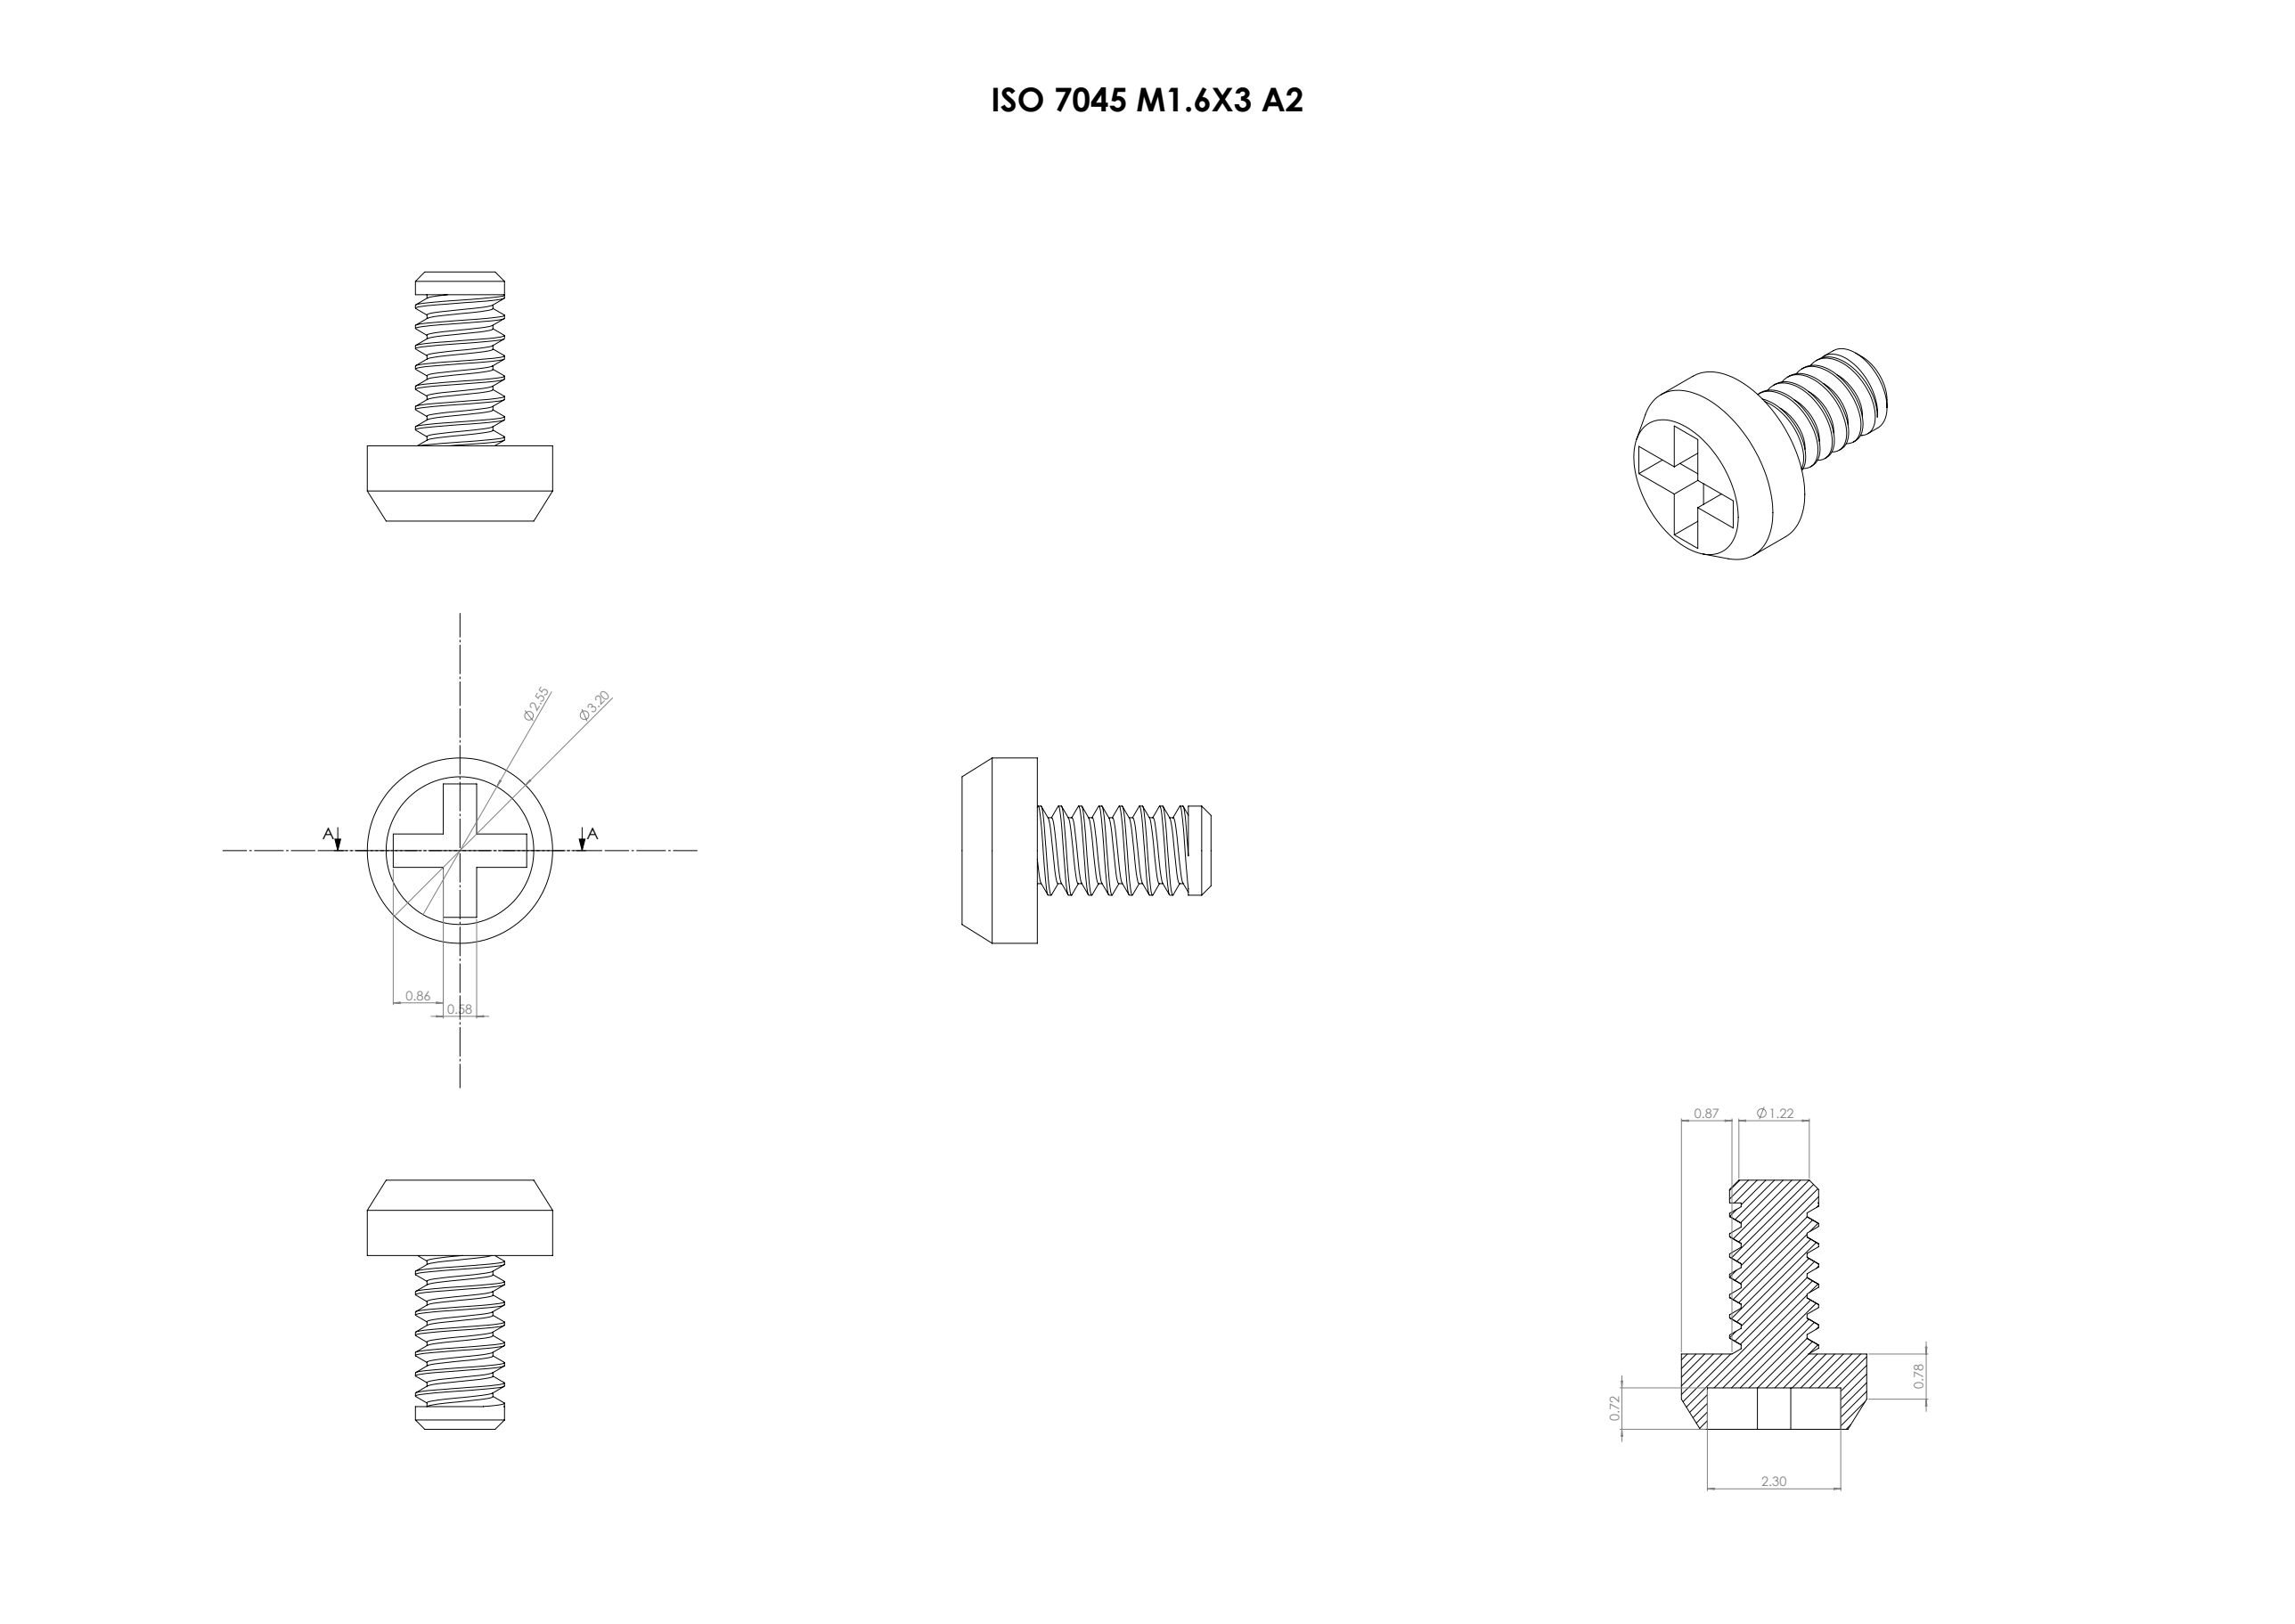
ISO-10303-21;
HEADER;
/* Generated by software containing ST-Developer
 * from STEP Tools, Inc. (www.steptools.com) 
 */

FILE_DESCRIPTION(
/* description */ (''),
/* implementation_level */ '2;1');

FILE_NAME(
/* name */ '18_ISO_7045_M1.6x3_A2.step',
/* time_stamp */ '2026-10-19T23:00:43-07:00',
/* author */ (''),
/* organization */ (''),
/* preprocessor_version */ 'ST-DEVELOPER v20.2',
/* originating_system */ 'Autodesk Translation Framework v15.15.0.0',
/* authorisation */ '');

FILE_SCHEMA (('AUTOMOTIVE_DESIGN { 1 0 10303 214 3 1 1 }'));
ENDSEC;

DATA;
#10=MECHANICAL_DESIGN_GEOMETRIC_PRESENTATION_REPRESENTATION('',(#1014),#55002);
#480=B_SPLINE_SURFACE_WITH_KNOTS('',3,3,((#51812,#51813,#51814,#51815,#51816,
#51817,#51818,#51819,#51820,#51821,#51822,#51823,#51824,#51825,#51826,#51827,
#51828,#51829,#51830,#51831,#51832,#51833,#51834,#51835,#51836,#51837,#51838,
#51839,#51840,#51841,#51842,#51843,#51844,#51845,#51846,#51847,#51848,#51849,
#51850,#51851,#51852,#51853,#51854,#51855,#51856,#51857,#51858,#51859,#51860,
#51861,#51862,#51863),(#51864,#51865,#51866,#51867,#51868,#51869,#51870,
#51871,#51872,#51873,#51874,#51875,#51876,#51877,#51878,#51879,#51880,#51881,
#51882,#51883,#51884,#51885,#51886,#51887,#51888,#51889,#51890,#51891,#51892,
#51893,#51894,#51895,#51896,#51897,#51898,#51899,#51900,#51901,#51902,#51903,
#51904,#51905,#51906,#51907,#51908,#51909,#51910,#51911,#51912,#51913,#51914,
#51915),(#51916,#51917,#51918,#51919,#51920,#51921,#51922,#51923,#51924,
#51925,#51926,#51927,#51928,#51929,#51930,#51931,#51932,#51933,#51934,#51935,
#51936,#51937,#51938,#51939,#51940,#51941,#51942,#51943,#51944,#51945,#51946,
#51947,#51948,#51949,#51950,#51951,#51952,#51953,#51954,#51955,#51956,#51957,
#51958,#51959,#51960,#51961,#51962,#51963,#51964,#51965,#51966,#51967),
(#51968,#51969,#51970,#51971,#51972,#51973,#51974,#51975,#51976,#51977,
#51978,#51979,#51980,#51981,#51982,#51983,#51984,#51985,#51986,#51987,#51988,
#51989,#51990,#51991,#51992,#51993,#51994,#51995,#51996,#51997,#51998,#51999,
#52000,#52001,#52002,#52003,#52004,#52005,#52006,#52007,#52008,#52009,#52010,
#52011,#52012,#52013,#52014,#52015,#52016,#52017,#52018,#52019)),
 .UNSPECIFIED.,.F.,.F.,.F.,(4,4),(4,1,1,1,1,1,1,1,1,1,1,1,1,1,1,1,1,1,1,
1,1,1,1,1,1,1,1,1,1,1,1,1,1,1,1,1,1,1,1,1,1,1,1,1,1,1,1,1,1,4),(0.,0.023094010767585),
(12.4478189520753,13.4456071169044,14.4433952817334,15.4411834465625,16.4389716113915,
17.4367597762206,18.4345479410496,19.4323361058786,20.4301242707077,21.4279124355367,
22.4257006003658,23.4234887651948,24.4212769300238,25.4190650948529,26.4168532596819,
27.414641424511,28.41242958934,29.410217754169,30.4080059189981,31.4057940838271,
32.4035822486562,33.4013704134852,34.3991585783142,35.3969467431433,36.3947349079723,
37.3925230728014,38.3903112376304,39.3880994024594,40.3858875672885,41.3836757321175,
42.3814638969466,43.3792520617756,44.3770402266046,45.3748283914337,46.3726165562627,
47.3704047210918,48.3681928859208,49.3659810507499,50.3637692155789,51.3615573804079,
52.359345545237,53.357133710066,54.3549218748951,55.3527100397241,56.3504982045531,
57.3482863693822,58.3460745342112,59.3438626990403,60.3416508638693,61.3394390286984),
 .UNSPECIFIED.);
#481=B_SPLINE_SURFACE_WITH_KNOTS('',3,3,((#52187,#52188,#52189,#52190,#52191,
#52192,#52193,#52194,#52195,#52196,#52197,#52198,#52199,#52200,#52201,#52202,
#52203,#52204,#52205,#52206,#52207,#52208,#52209,#52210,#52211,#52212,#52213,
#52214,#52215,#52216,#52217,#52218,#52219,#52220,#52221,#52222,#52223,#52224,
#52225,#52226,#52227,#52228,#52229,#52230,#52231,#52232,#52233,#52234,#52235,
#52236,#52237,#52238),(#52239,#52240,#52241,#52242,#52243,#52244,#52245,
#52246,#52247,#52248,#52249,#52250,#52251,#52252,#52253,#52254,#52255,#52256,
#52257,#52258,#52259,#52260,#52261,#52262,#52263,#52264,#52265,#52266,#52267,
#52268,#52269,#52270,#52271,#52272,#52273,#52274,#52275,#52276,#52277,#52278,
#52279,#52280,#52281,#52282,#52283,#52284,#52285,#52286,#52287,#52288,#52289,
#52290),(#52291,#52292,#52293,#52294,#52295,#52296,#52297,#52298,#52299,
#52300,#52301,#52302,#52303,#52304,#52305,#52306,#52307,#52308,#52309,#52310,
#52311,#52312,#52313,#52314,#52315,#52316,#52317,#52318,#52319,#52320,#52321,
#52322,#52323,#52324,#52325,#52326,#52327,#52328,#52329,#52330,#52331,#52332,
#52333,#52334,#52335,#52336,#52337,#52338,#52339,#52340,#52341,#52342),
(#52343,#52344,#52345,#52346,#52347,#52348,#52349,#52350,#52351,#52352,
#52353,#52354,#52355,#52356,#52357,#52358,#52359,#52360,#52361,#52362,#52363,
#52364,#52365,#52366,#52367,#52368,#52369,#52370,#52371,#52372,#52373,#52374,
#52375,#52376,#52377,#52378,#52379,#52380,#52381,#52382,#52383,#52384,#52385,
#52386,#52387,#52388,#52389,#52390,#52391,#52392,#52393,#52394)),
 .UNSPECIFIED.,.F.,.F.,.F.,(4,4),(4,1,1,1,1,1,1,1,1,1,1,1,1,1,1,1,1,1,1,
1,1,1,1,1,1,1,1,1,1,1,1,1,1,1,1,1,1,1,1,1,1,1,1,1,1,1,1,1,1,4),(0.,0.023094010767585),
(15.7552446903951,16.7530328552242,17.7508210200532,18.7486091848822,19.7463973497113,
20.7441855145403,21.7419736793694,22.7397618441984,23.7375500090275,24.7353381738565,
25.7331263386855,26.7309145035146,27.7287026683436,28.7264908331727,29.7242789980017,
30.7220671628307,31.7198553276598,32.7176434924888,33.7154316573179,34.7132198221469,
35.7110079869759,36.708796151805,37.706584316634,38.7043724814631,39.7021606462921,
40.6999488111211,41.6977369759502,42.6955251407792,43.6933133056083,44.6911014704373,
45.6888896352663,46.6866778000954,47.6844659649244,48.6822541297535,49.6800422945825,
50.6778304594116,51.6756186242406,52.6734067890696,53.6711949538987,54.6689831187277,
55.6667712835568,56.6645594483858,57.6623476132148,58.6601357780439,59.6579239428729,
60.655712107702,61.653500272531,62.6512884373601,63.6490766021891,64.6468647670181),
 .UNSPECIFIED.);
#845=B_SPLINE_CURVE_WITH_KNOTS('',3,(#51284,#51285,#51286,#51287,#51288,
#51289,#51290,#51291,#51292,#51293,#51294,#51295,#51296,#51297,#51298,#51299),
 .UNSPECIFIED.,.F.,.F.,(4,3,3,3,3,4),(-6.2359038847334,-5.98672898897424,
-4.9889408241452,-3.99115265931616,-2.99336449448712,-2.07291355912483),
 .UNSPECIFIED.);
#846=B_SPLINE_CURVE_WITH_KNOTS('',3,(#51307,#51308,#51309,#51310,#51311,
#51312,#51313,#51314,#51315,#51316,#51317,#51318,#51319),.UNSPECIFIED.,
 .F.,.F.,(4,3,3,3,4),(0.,0.997788164829036,1.99557632965808,2.99336449448712,
3.26014431587357),.UNSPECIFIED.);
#847=B_SPLINE_CURVE_WITH_KNOTS('',3,(#51324,#51325,#51326,#51327,#51328,
#51329,#51330,#51331,#51332,#51333,#51334,#51335,#51336,#51337,#51338,#51339,
#51340,#51341,#51342,#51343,#51344,#51345),.UNSPECIFIED.,.F.,.F.,(4,3,3,
3,3,3,3,4),(-12.519089191913,-11.9734579779485,-10.9756698131195,-9.97788164829041,
-8.98009348346137,-7.98230531863233,-6.98451715380329,-6.2359038847334),
 .UNSPECIFIED.);
#848=B_SPLINE_CURVE_WITH_KNOTS('',3,(#51346,#51347,#51348,#51349,#51350,
#51351,#51352,#51353,#51354,#51355,#51356,#51357,#51358,#51359,#51360,#51361,
#51362,#51363,#51364,#51365,#51366,#51367),.UNSPECIFIED.,.F.,.F.,(4,3,3,
3,3,3,3,4),(3.26014431587357,3.99115265931617,4.9889408241452,5.98672898897425,
6.98451715380329,7.98230531863232,8.98009348346137,9.54332962305316),
 .UNSPECIFIED.);
#849=B_SPLINE_CURVE_WITH_KNOTS('',3,(#51372,#51373,#51374,#51375,#51376,
#51377,#51378,#51379,#51380,#51381,#51382,#51383,#51384,#51385,#51386,#51387,
#51388,#51389,#51390,#51391,#51392,#51393),.UNSPECIFIED.,.F.,.F.,(4,3,3,
3,3,3,3,4),(-18.8022744990926,-17.9601869669227,-16.9623988020937,-15.9646106372647,
-14.9668224724356,-13.9690343076066,-12.9712461427775,-12.519089191913),
 .UNSPECIFIED.);
#850=B_SPLINE_CURVE_WITH_KNOTS('',3,(#51394,#51395,#51396,#51397,#51398,
#51399,#51400,#51401,#51402,#51403,#51404,#51405,#51406,#51407,#51408,#51409,
#51410,#51411,#51412,#51413,#51414,#51415),.UNSPECIFIED.,.F.,.F.,(4,3,3,
3,3,3,3,4),(9.54332962305316,9.97788164829041,10.9756698131194,11.9734579779485,
12.9712461427775,13.9690343076066,14.9668224724356,15.8265149302327),
 .UNSPECIFIED.);
#851=B_SPLINE_CURVE_WITH_KNOTS('',3,(#51420,#51421,#51422,#51423,#51424,
#51425,#51426,#51427,#51428,#51429,#51430,#51431,#51432,#51433,#51434,#51435,
#51436,#51437,#51438,#51439,#51440,#51441,#51442,#51443,#51444),
 .UNSPECIFIED.,.F.,.F.,(4,3,3,3,3,3,3,3,4),(-25.0854598062722,-24.944704120726,
-23.946915955897,-22.9491277910679,-21.9513396262389,-20.9535514614099,
-19.9557632965808,-18.9579751317518,-18.8022744990926),.UNSPECIFIED.);
#852=B_SPLINE_CURVE_WITH_KNOTS('',3,(#51445,#51446,#51447,#51448,#51449,
#51450,#51451,#51452,#51453,#51454,#51455,#51456,#51457,#51458,#51459,#51460,
#51461,#51462,#51463,#51464,#51465,#51466,#51467,#51468,#51469),
 .UNSPECIFIED.,.F.,.F.,(4,3,3,3,3,3,3,3,4),(15.8265149302327,15.9646106372647,
16.9623988020937,17.9601869669227,18.9579751317518,19.9557632965808,20.9535514614099,
21.9513396262389,22.1097002374123),.UNSPECIFIED.);
#853=B_SPLINE_CURVE_WITH_KNOTS('',3,(#51474,#51475,#51476,#51477,#51478,
#51479,#51480,#51481,#51482,#51483,#51484,#51485,#51486,#51487,#51488,#51489,
#51490,#51491,#51492,#51493,#51494,#51495),.UNSPECIFIED.,.F.,.F.,(4,3,3,
3,3,3,3,4),(-31.3686451134517,-30.9314331097003,-29.9336449448712,-28.9358567800422,
-27.9380686152131,-26.9402804503841,-25.9424922855551,-25.0854598062722),
 .UNSPECIFIED.);
#854=B_SPLINE_CURVE_WITH_KNOTS('',3,(#51496,#51497,#51498,#51499,#51500,
#51501,#51502,#51503,#51504,#51505,#51506,#51507,#51508,#51509,#51510,#51511,
#51512,#51513,#51514,#51515,#51516,#51517),.UNSPECIFIED.,.F.,.F.,(4,3,3,
3,3,3,3,4),(22.1097002374123,22.9491277910679,23.946915955897,24.944704120726,
25.9424922855551,26.9402804503841,27.9380686152131,28.3928855445919),
 .UNSPECIFIED.);
#855=B_SPLINE_CURVE_WITH_KNOTS('',3,(#51522,#51523,#51524,#51525,#51526,
#51527,#51528,#51529,#51530,#51531,#51532,#51533,#51534,#51535,#51536,#51537,
#51538,#51539,#51540,#51541,#51542,#51543),.UNSPECIFIED.,.F.,.F.,(4,3,3,
3,3,3,3,4),(-37.6518304206313,-36.9181620986745,-35.9203739338455,-34.9225857690164,
-33.9247976041874,-32.9270094393584,-31.9292212745293,-31.3686451134517),
 .UNSPECIFIED.);
#856=B_SPLINE_CURVE_WITH_KNOTS('',3,(#51544,#51545,#51546,#51547,#51548,
#51549,#51550,#51551,#51552,#51553,#51554,#51555,#51556,#51557,#51558,#51559,
#51560,#51561,#51562,#51563,#51564,#51565),.UNSPECIFIED.,.F.,.F.,(4,3,3,
3,3,3,3,4),(28.3928855445919,28.9358567800422,29.9336449448712,30.9314331097003,
31.9292212745293,32.9270094393584,33.9247976041874,34.6760708517715),
 .UNSPECIFIED.);
#857=B_SPLINE_CURVE_WITH_KNOTS('',3,(#51570,#51571,#51572,#51573,#51574,
#51575,#51576,#51577,#51578,#51579,#51580,#51581,#51582,#51583,#51584,#51585,
#51586,#51587,#51588,#51589,#51590,#51591,#51592,#51593,#51594),
 .UNSPECIFIED.,.F.,.F.,(4,3,3,3,3,3,3,3,4),(-43.9350157278109,-43.9026792524778,
-42.9048910876488,-41.9071029228197,-40.9093147579907,-39.9115265931616,
-38.9137384283326,-37.9159502635036,-37.6518304206313),.UNSPECIFIED.);
#858=B_SPLINE_CURVE_WITH_KNOTS('',3,(#51595,#51596,#51597,#51598,#51599,
#51600,#51601,#51602,#51603,#51604,#51605,#51606,#51607,#51608,#51609,#51610,
#51611,#51612,#51613,#51614,#51615,#51616,#51617,#51618,#51619),
 .UNSPECIFIED.,.F.,.F.,(4,3,3,3,3,3,3,3,4),(34.6760708517715,34.9225857690164,
35.9203739338455,36.9181620986745,37.9159502635036,38.9137384283326,39.9115265931616,
40.9093147579907,40.9592561589511),.UNSPECIFIED.);
#859=B_SPLINE_CURVE_WITH_KNOTS('',3,(#51625,#51626,#51627,#51628,#51629,
#51630),.UNSPECIFIED.,.F.,.F.,(4,1,1,4),(59.6902604182061,60.655712107702,
61.653500272531,62.5739512078933),.UNSPECIFIED.);
#860=B_SPLINE_CURVE_WITH_KNOTS('',3,(#51633,#51634,#51635,#51636,#51637),
 .UNSPECIFIED.,.F.,.F.,(4,1,4),(59.6902604182061,60.3416508638693,61.3394390286984),
 .UNSPECIFIED.);
#861=B_SPLINE_CURVE_WITH_KNOTS('',3,(#51642,#51643,#51644,#51645,#51646,
#51647,#51648,#51649,#51650,#51651,#51652),.UNSPECIFIED.,.F.,.F.,(4,1,1,
1,1,1,1,1,4),(53.4070751110265,53.6711949538987,54.6689831187277,55.6667712835568,
56.6645594483858,57.6623476132148,58.6601357780439,59.6579239428729,59.6902604182061),
 .UNSPECIFIED.);
#862=B_SPLINE_CURVE_WITH_KNOTS('',3,(#51653,#51654,#51655,#51656,#51657,
#51658,#51659,#51660,#51661,#51662),.UNSPECIFIED.,.F.,.F.,(4,1,1,1,1,1,
1,4),(53.4070751110265,54.3549218748951,55.3527100397241,56.3504982045531,
57.3482863693822,58.3460745342112,59.3438626990403,59.6902604182061),
 .UNSPECIFIED.);
#863=B_SPLINE_CURVE_WITH_KNOTS('',3,(#51667,#51668,#51669,#51670,#51671,
#51672,#51673,#51674,#51675,#51676),.UNSPECIFIED.,.F.,.F.,(4,1,1,1,1,1,
1,4),(47.1238898038469,47.6844659649244,48.6822541297535,49.6800422945825,
50.6778304594116,51.6756186242406,52.6734067890696,53.4070751110265),
 .UNSPECIFIED.);
#864=B_SPLINE_CURVE_WITH_KNOTS('',3,(#51677,#51678,#51679,#51680,#51681,
#51682,#51683,#51684,#51685,#51686,#51687),.UNSPECIFIED.,.F.,.F.,(4,1,1,
1,1,1,1,1,4),(47.1238898038469,47.3704047210918,48.3681928859208,49.3659810507499,
50.3637692155789,51.3615573804079,52.359345545237,53.357133710066,53.4070751110265),
 .UNSPECIFIED.);
#865=B_SPLINE_CURVE_WITH_KNOTS('',3,(#51692,#51693,#51694,#51695,#51696,
#51697,#51698,#51699,#51700,#51701),.UNSPECIFIED.,.F.,.F.,(4,1,1,1,1,1,
1,4),(40.8407044966673,41.6977369759502,42.6955251407792,43.6933133056083,
44.6911014704373,45.6888896352663,46.6866778000954,47.1238898038469),
 .UNSPECIFIED.);
#866=B_SPLINE_CURVE_WITH_KNOTS('',3,(#51702,#51703,#51704,#51705,#51706,
#51707,#51708,#51709,#51710,#51711),.UNSPECIFIED.,.F.,.F.,(4,1,1,1,1,1,
1,4),(40.8407044966673,41.3836757321175,42.3814638969466,43.3792520617756,
44.3770402266046,45.3748283914337,46.3726165562627,47.1238898038469),
 .UNSPECIFIED.);
#867=B_SPLINE_CURVE_WITH_KNOTS('',3,(#51716,#51717,#51718,#51719,#51720,
#51721,#51722,#51723,#51724,#51725,#51726),.UNSPECIFIED.,.F.,.F.,(4,1,1,
1,1,1,1,1,4),(34.5575191894877,34.7132198221469,35.7110079869759,36.708796151805,
37.706584316634,38.7043724814631,39.7021606462921,40.6999488111211,40.8407044966673),
 .UNSPECIFIED.);
#868=B_SPLINE_CURVE_WITH_KNOTS('',3,(#51727,#51728,#51729,#51730,#51731,
#51732,#51733,#51734,#51735,#51736),.UNSPECIFIED.,.F.,.F.,(4,1,1,1,1,1,
1,4),(34.5575191894877,35.3969467431433,36.3947349079723,37.3925230728014,
38.3903112376304,39.3880994024594,40.3858875672885,40.8407044966673),
 .UNSPECIFIED.);
#869=B_SPLINE_CURVE_WITH_KNOTS('',3,(#51741,#51742,#51743,#51744,#51745,
#51746,#51747,#51748,#51749,#51750),.UNSPECIFIED.,.F.,.F.,(4,1,1,1,1,1,
1,4),(28.2743338823081,28.7264908331727,29.7242789980017,30.7220671628307,
31.7198553276598,32.7176434924888,33.7154316573179,34.5575191894877),
 .UNSPECIFIED.);
#870=B_SPLINE_CURVE_WITH_KNOTS('',3,(#51751,#51752,#51753,#51754,#51755,
#51756,#51757,#51758,#51759,#51760,#51761),.UNSPECIFIED.,.F.,.F.,(4,1,1,
1,1,1,1,1,4),(28.2743338823081,28.41242958934,29.410217754169,30.4080059189981,
31.4057940838271,32.4035822486562,33.4013704134852,34.3991585783142,34.5575191894877),
 .UNSPECIFIED.);
#871=B_SPLINE_CURVE_WITH_KNOTS('',3,(#51766,#51767,#51768,#51769,#51770,
#51771,#51772,#51773,#51774,#51775),.UNSPECIFIED.,.F.,.F.,(4,1,1,1,1,1,
1,4),(21.9911485751285,22.7397618441984,23.7375500090275,24.7353381738565,
25.7331263386855,26.7309145035146,27.7287026683436,28.2743338823081),
 .UNSPECIFIED.);
#872=B_SPLINE_CURVE_WITH_KNOTS('',3,(#51776,#51777,#51778,#51779,#51780,
#51781,#51782,#51783,#51784,#51785),.UNSPECIFIED.,.F.,.F.,(4,1,1,1,1,1,
1,4),(21.9911485751285,22.4257006003658,23.4234887651948,24.4212769300238,
25.4190650948529,26.4168532596819,27.414641424511,28.2743338823081),
 .UNSPECIFIED.);
#873=B_SPLINE_CURVE_WITH_KNOTS('',3,(#51792,#51793,#51794,#51795,#51796,
#51797,#51798,#51799,#51800,#51801),.UNSPECIFIED.,.F.,.F.,(4,1,1,1,1,1,
1,4),(15.7552446903951,16.7530328552242,17.7508210200532,18.7486091848822,
19.7463973497113,20.7441855145403,21.7419736793694,21.9911485751285),
 .UNSPECIFIED.);
#874=B_SPLINE_CURVE_WITH_KNOTS('',3,(#51802,#51803,#51804,#51805,#51806,
#51807,#51808,#51809,#51810,#51811),.UNSPECIFIED.,.F.,.F.,(4,1,1,1,1,1,
1,4),(15.7079632679489,16.4389716113915,17.4367597762206,18.4345479410496,
19.4323361058786,20.4301242707077,21.4279124355367,21.9911485751285),
 .UNSPECIFIED.);
#875=B_SPLINE_CURVE_WITH_KNOTS('',3,(#52021,#52022,#52023,#52024,#52025,
#52026,#52027,#52028,#52029,#52030,#52031,#52032,#52033,#52034,#52035,#52036,
#52037,#52038,#52039,#52040,#52041,#52042,#52043,#52044,#52045,#52046,#52047,
#52048,#52049,#52050,#52051,#52052,#52053,#52054,#52055,#52056,#52057,#52058,
#52059,#52060,#52061,#52062,#52063,#52064,#52065,#52066),.UNSPECIFIED.,
 .F.,.F.,(4,3,3,3,3,3,3,3,3,3,3,3,3,3,3,4),(-0.140062757837278,-0.134123173823536,
-0.121523401165327,-0.113447705434834,-0.0990655075399137,-0.0919518085532341,
-0.0750566738033047,-0.0674043852357639,-0.0624390856721942,-0.0527351001118668,
-0.0459772985974198,-0.0296762170335496,-0.0230583683643434,-0.016477620433628,
-0.00151411940223995,0.),.UNSPECIFIED.);
#876=B_SPLINE_CURVE_WITH_KNOTS('',3,(#52067,#52068,#52069,#52070,#52071,
#52072,#52073,#52074,#52075,#52076,#52077,#52078,#52079,#52080,#52081,#52082,
#52083,#52084,#52085),.UNSPECIFIED.,.F.,.F.,(4,3,3,3,3,3,4),(40.9592561589511,
41.9071029228197,42.9048910876487,43.9026792524778,44.9004674173068,45.8982555821359,
46.8187065174982),.UNSPECIFIED.);
#877=B_SPLINE_CURVE_WITH_KNOTS('',3,(#52087,#52088,#52089,#52090,#52091,
#52092,#52093,#52094,#52095,#52096,#52097,#52098,#52099,#52100,#52101,#52102,
#52103,#52104,#52105,#52106,#52107,#52108,#52109,#52110,#52111,#52112,#52113,
#52114,#52115,#52116,#52117,#52118,#52119,#52120,#52121,#52122,#52123,#52124,
#52125,#52126,#52127,#52128,#52129,#52130,#52131,#52132),.UNSPECIFIED.,
 .F.,.F.,(4,3,3,3,3,3,3,3,3,3,3,3,3,3,3,4),(-0.140969988491048,-0.136446439322258,
-0.126660801898424,-0.119269074856758,-0.10953502353942,-0.102598331591438,
-0.0857596038079746,-0.0787758183049045,-0.072931898136125,-0.0587706520901876,
-0.0520483890707233,-0.0380705861802498,-0.0301255169382023,-0.023298848983932,
-0.00434997386540177,0.),.UNSPECIFIED.);
#878=B_SPLINE_CURVE_WITH_KNOTS('',3,(#52133,#52134,#52135,#52136,#52137),
 .UNSPECIFIED.,.F.,.F.,(4,1,4),(14.5207325112002,15.4411834465625,15.7079632679489),
 .UNSPECIFIED.);
#879=B_SPLINE_CURVE_WITH_KNOTS('',3,(#52139,#52140,#52141,#52142,#52143,
#52144,#52145,#52146,#52147,#52148,#52149,#52150,#52151,#52152,#52153,#52154,
#52155,#52156,#52157,#52158,#52159,#52160,#52161,#52162,#52163,#52164,#52165,
#52166,#52167,#52168,#52169,#52170,#52171,#52172,#52173,#52174,#52175,#52176,
#52177,#52178,#52179,#52180,#52181,#52182,#52183,#52184),.UNSPECIFIED.,
 .F.,.F.,(4,3,3,3,3,3,3,3,3,3,3,3,3,3,3,4),(-0.140062757837251,-0.134123173823509,
-0.121523399045325,-0.11344770204781,-0.0990654838477444,-0.0919518011861085,
-0.0750566620112235,-0.0674043807182989,-0.062439085672185,-0.0527351170922762,
-0.0459772905666743,-0.029676213594428,-0.0230583524982984,-0.0164776174494443,
-0.00151412549618594,0.),.UNSPECIFIED.);
#880=B_SPLINE_CURVE_WITH_KNOTS('',3,(#52396,#52397,#52398,#52399,#52400,
#52401,#52402,#52403,#52404,#52405,#52406,#52407,#52408,#52409,#52410,#52411,
#52412,#52413,#52414,#52415,#52416,#52417,#52418,#52419,#52420,#52421,#52422,
#52423,#52424,#52425,#52426,#52427,#52428,#52429,#52430,#52431,#52432,#52433,
#52434,#52435,#52436,#52437,#52438,#52439,#52440,#52441),.UNSPECIFIED.,
 .F.,.F.,(4,3,3,3,3,3,3,3,3,3,3,3,3,3,3,4),(-0.140969988491049,-0.136446439322259,
-0.126660808831101,-0.11926908034975,-0.109535054430385,-0.102598368559059,
-0.0857596411563137,-0.0787758156854511,-0.0729318981361281,-0.0587706585020556,
-0.0520483951910087,-0.0380705929416598,-0.030125518229324,-0.0232988520606989,
-0.00434997944539849,0.),.UNSPECIFIED.);
#881=B_SPLINE_CURVE_WITH_KNOTS('',3,(#52442,#52443,#52444,#52445,#52446,
#52447,#52448,#52449,#52450,#52451,#52452,#52453,#52454,#52455,#52456,#52457),
 .UNSPECIFIED.,.F.,.F.,(4,3,3,3,3,4),(-48.891620076623,-47.893831911794,
-46.8960437469649,-45.8982555821359,-44.9004674173068,-43.9350157278109),
 .UNSPECIFIED.);
#974=SHAPE_REPRESENTATION_RELATIONSHIP('SRR','None',#55122,#994);
#994=ADVANCED_BREP_SHAPE_REPRESENTATION('',(#1034),#55000);
#1014=STYLED_ITEM('',(#55400),#1034);
#1034=MANIFOLD_SOLID_BREP('ISO_7045_M1.6x3_A2',#24547);
#1272=FACE_BOUND('',#5306,.T.);
#1273=FACE_BOUND('',#5318,.T.);
#1918=PLANE('',#27046);
#1919=PLANE('',#27049);
#1920=PLANE('',#27050);
#1921=PLANE('',#27051);
#1922=PLANE('',#27052);
#1923=PLANE('',#27053);
#1924=PLANE('',#27054);
#1925=PLANE('',#27055);
#1926=PLANE('',#27057);
#1927=PLANE('',#27058);
#1928=PLANE('',#27059);
#1929=PLANE('',#27060);
#1930=PLANE('',#27061);
#1931=PLANE('',#27062);
#1932=PLANE('',#27063);
#1933=PLANE('',#27064);
#1934=PLANE('',#27069);
#2358=CYLINDRICAL_SURFACE('',#27026,0.076925);
#2359=CYLINDRICAL_SURFACE('',#27030,0.076925);
#2360=CYLINDRICAL_SURFACE('',#27031,0.076925);
#2361=CYLINDRICAL_SURFACE('',#27032,0.076925);
#2362=CYLINDRICAL_SURFACE('',#27033,0.076925);
#2363=CYLINDRICAL_SURFACE('',#27034,0.076925);
#2364=CYLINDRICAL_SURFACE('',#27035,0.076925);
#2365=CYLINDRICAL_SURFACE('',#27036,0.056925);
#2366=CYLINDRICAL_SURFACE('',#27038,0.056925);
#2367=CYLINDRICAL_SURFACE('',#27039,0.056925);
#2368=CYLINDRICAL_SURFACE('',#27040,0.056925);
#2369=CYLINDRICAL_SURFACE('',#27041,0.056925);
#2370=CYLINDRICAL_SURFACE('',#27042,0.056925);
#2371=CYLINDRICAL_SURFACE('',#27043,0.056925);
#2372=CYLINDRICAL_SURFACE('',#27044,0.056925);
#2373=CYLINDRICAL_SURFACE('',#27048,0.056925);
#2374=CYLINDRICAL_SURFACE('',#27067,0.076925);
#2375=CYLINDRICAL_SURFACE('',#27071,0.16);
#3680=FACE_OUTER_BOUND('',#5280,.T.);
#3681=FACE_OUTER_BOUND('',#5281,.T.);
#3682=FACE_OUTER_BOUND('',#5282,.T.);
#3683=FACE_OUTER_BOUND('',#5283,.T.);
#3684=FACE_OUTER_BOUND('',#5284,.T.);
#3685=FACE_OUTER_BOUND('',#5285,.T.);
#3686=FACE_OUTER_BOUND('',#5286,.T.);
#3687=FACE_OUTER_BOUND('',#5287,.T.);
#3688=FACE_OUTER_BOUND('',#5288,.T.);
#3689=FACE_OUTER_BOUND('',#5289,.T.);
#3690=FACE_OUTER_BOUND('',#5290,.T.);
#3691=FACE_OUTER_BOUND('',#5291,.T.);
#3692=FACE_OUTER_BOUND('',#5292,.T.);
#3693=FACE_OUTER_BOUND('',#5293,.T.);
#3694=FACE_OUTER_BOUND('',#5294,.T.);
#3695=FACE_OUTER_BOUND('',#5295,.T.);
#3696=FACE_OUTER_BOUND('',#5296,.T.);
#3697=FACE_OUTER_BOUND('',#5297,.T.);
#3698=FACE_OUTER_BOUND('',#5298,.T.);
#3699=FACE_OUTER_BOUND('',#5299,.T.);
#3700=FACE_OUTER_BOUND('',#5300,.T.);
#3701=FACE_OUTER_BOUND('',#5301,.T.);
#3702=FACE_OUTER_BOUND('',#5302,.T.);
#3703=FACE_OUTER_BOUND('',#5303,.T.);
#3704=FACE_OUTER_BOUND('',#5304,.T.);
#3705=FACE_OUTER_BOUND('',#5305,.T.);
#3706=FACE_OUTER_BOUND('',#5307,.T.);
#3707=FACE_OUTER_BOUND('',#5308,.T.);
#3708=FACE_OUTER_BOUND('',#5309,.T.);
#3709=FACE_OUTER_BOUND('',#5310,.T.);
#3710=FACE_OUTER_BOUND('',#5311,.T.);
#3711=FACE_OUTER_BOUND('',#5312,.T.);
#3712=FACE_OUTER_BOUND('',#5313,.T.);
#3713=FACE_OUTER_BOUND('',#5314,.T.);
#3714=FACE_OUTER_BOUND('',#5315,.T.);
#3715=FACE_OUTER_BOUND('',#5316,.T.);
#3716=FACE_OUTER_BOUND('',#5317,.T.);
#3717=FACE_OUTER_BOUND('',#5319,.T.);
#3718=FACE_OUTER_BOUND('',#5320,.T.);
#5280=EDGE_LOOP('',(#22436,#22437,#22438,#22439,#22440,#22441,#22442,#22443));
#5281=EDGE_LOOP('',(#22444,#22445,#22446,#22447));
#5282=EDGE_LOOP('',(#22448,#22449,#22450,#22451));
#5283=EDGE_LOOP('',(#22452,#22453,#22454,#22455));
#5284=EDGE_LOOP('',(#22456,#22457,#22458,#22459));
#5285=EDGE_LOOP('',(#22460,#22461,#22462,#22463));
#5286=EDGE_LOOP('',(#22464,#22465,#22466,#22467));
#5287=EDGE_LOOP('',(#22468,#22469,#22470,#22471));
#5288=EDGE_LOOP('',(#22472,#22473,#22474,#22475));
#5289=EDGE_LOOP('',(#22476,#22477,#22478,#22479));
#5290=EDGE_LOOP('',(#22480,#22481,#22482,#22483));
#5291=EDGE_LOOP('',(#22484,#22485,#22486,#22487));
#5292=EDGE_LOOP('',(#22488,#22489,#22490,#22491));
#5293=EDGE_LOOP('',(#22492,#22493,#22494,#22495));
#5294=EDGE_LOOP('',(#22496,#22497,#22498,#22499,#22500));
#5295=EDGE_LOOP('',(#22501,#22502,#22503,#22504,#22505,#22506,#22507,#22508,
#22509,#22510,#22511,#22512,#22513,#22514,#22515,#22516,#22517,#22518,#22519));
#5296=EDGE_LOOP('',(#22520,#22521,#22522,#22523,#22524,#22525));
#5297=EDGE_LOOP('',(#22526,#22527,#22528));
#5298=EDGE_LOOP('',(#22529,#22530,#22531,#22532,#22533,#22534,#22535,#22536,
#22537,#22538,#22539,#22540,#22541,#22542,#22543,#22544,#22545,#22546));
#5299=EDGE_LOOP('',(#22547,#22548,#22549,#22550));
#5300=EDGE_LOOP('',(#22551,#22552,#22553,#22554));
#5301=EDGE_LOOP('',(#22555,#22556,#22557,#22558));
#5302=EDGE_LOOP('',(#22559,#22560,#22561,#22562));
#5303=EDGE_LOOP('',(#22563,#22564,#22565,#22566));
#5304=EDGE_LOOP('',(#22567,#22568,#22569,#22570));
#5305=EDGE_LOOP('',(#22571));
#5306=EDGE_LOOP('',(#22572,#22573,#22574,#22575,#22576,#22577,#22578,#22579,
#22580,#22581,#22582,#22583));
#5307=EDGE_LOOP('',(#22584,#22585,#22586,#22587));
#5308=EDGE_LOOP('',(#22588,#22589,#22590,#22591));
#5309=EDGE_LOOP('',(#22592,#22593,#22594,#22595));
#5310=EDGE_LOOP('',(#22596,#22597,#22598,#22599));
#5311=EDGE_LOOP('',(#22600,#22601,#22602,#22603));
#5312=EDGE_LOOP('',(#22604,#22605,#22606,#22607));
#5313=EDGE_LOOP('',(#22608,#22609,#22610,#22611,#22612,#22613,#22614,#22615,
#22616,#22617,#22618,#22619));
#5314=EDGE_LOOP('',(#22620));
#5315=EDGE_LOOP('',(#22621,#22622,#22623,#22624));
#5316=EDGE_LOOP('',(#22625,#22626,#22627,#22628));
#5317=EDGE_LOOP('',(#22629));
#5318=EDGE_LOOP('',(#22630,#22631,#22632,#22633));
#5319=EDGE_LOOP('',(#22634,#22635,#22636,#22637));
#5320=EDGE_LOOP('',(#22638,#22639,#22640,#22641));
#7073=LINE('',#51282,#8894);
#7074=LINE('',#51303,#8895);
#7075=LINE('',#51323,#8896);
#7076=LINE('',#51371,#8897);
#7077=LINE('',#51419,#8898);
#7078=LINE('',#51473,#8899);
#7079=LINE('',#51521,#8900);
#7080=LINE('',#51569,#8901);
#7081=LINE('',#51623,#8902);
#7082=LINE('',#51641,#8903);
#7083=LINE('',#51666,#8904);
#7084=LINE('',#51691,#8905);
#7085=LINE('',#51715,#8906);
#7086=LINE('',#51740,#8907);
#7087=LINE('',#51765,#8908);
#7088=LINE('',#51789,#8909);
#7089=LINE('',#52461,#8910);
#7090=LINE('',#52463,#8911);
#7091=LINE('',#52465,#8912);
#7092=LINE('',#52466,#8913);
#7093=LINE('',#52470,#8914);
#7094=LINE('',#52472,#8915);
#7095=LINE('',#52474,#8916);
#7096=LINE('',#52475,#8917);
#7097=LINE('',#52479,#8918);
#7098=LINE('',#52481,#8919);
#7099=LINE('',#52483,#8920);
#7100=LINE('',#52484,#8921);
#7101=LINE('',#52487,#8922);
#7102=LINE('',#52489,#8923);
#7103=LINE('',#52490,#8924);
#7104=LINE('',#52492,#8925);
#7105=LINE('',#52493,#8926);
#7106=LINE('',#52496,#8927);
#7107=LINE('',#52498,#8928);
#7108=LINE('',#52499,#8929);
#7109=LINE('',#52504,#8930);
#7110=LINE('',#52506,#8931);
#7111=LINE('',#52507,#8932);
#7112=LINE('',#52509,#8933);
#7113=LINE('',#52511,#8934);
#7114=LINE('',#52512,#8935);
#7115=LINE('',#52515,#8936);
#7116=LINE('',#52516,#8937);
#7117=LINE('',#52519,#8938);
#7118=LINE('',#52520,#8939);
#7119=LINE('',#52523,#8940);
#7120=LINE('',#52524,#8941);
#7121=LINE('',#52527,#8942);
#7122=LINE('',#52528,#8943);
#7123=LINE('',#52530,#8944);
#7124=LINE('',#52532,#8945);
#7125=LINE('',#52538,#8946);
#7126=LINE('',#52547,#8947);
#7127=LINE('',#52549,#8948);
#8894=VECTOR('',#33403,0.08);
#8895=VECTOR('',#33406,0.08);
#8896=VECTOR('',#33413,0.08);
#8897=VECTOR('',#33416,0.08);
#8898=VECTOR('',#33419,0.08);
#8899=VECTOR('',#33422,0.08);
#8900=VECTOR('',#33425,0.08);
#8901=VECTOR('',#33428,0.08);
#8902=VECTOR('',#33431,0.056925);
#8903=VECTOR('',#33436,0.056925);
#8904=VECTOR('',#33439,0.056925);
#8905=VECTOR('',#33442,0.056925);
#8906=VECTOR('',#33445,0.056925);
#8907=VECTOR('',#33448,0.056925);
#8908=VECTOR('',#33451,0.056925);
#8909=VECTOR('',#33454,0.056925);
#8910=VECTOR('',#33465,1.);
#8911=VECTOR('',#33466,1.);
#8912=VECTOR('',#33467,1.);
#8913=VECTOR('',#33468,1.);
#8914=VECTOR('',#33471,1.);
#8915=VECTOR('',#33472,1.);
#8916=VECTOR('',#33473,1.);
#8917=VECTOR('',#33474,1.);
#8918=VECTOR('',#33477,1.);
#8919=VECTOR('',#33478,1.);
#8920=VECTOR('',#33479,1.);
#8921=VECTOR('',#33480,1.);
#8922=VECTOR('',#33483,1.);
#8923=VECTOR('',#33484,1.);
#8924=VECTOR('',#33485,1.);
#8925=VECTOR('',#33488,1.);
#8926=VECTOR('',#33489,1.);
#8927=VECTOR('',#33492,1.);
#8928=VECTOR('',#33493,1.);
#8929=VECTOR('',#33494,1.);
#8930=VECTOR('',#33499,1.);
#8931=VECTOR('',#33500,1.);
#8932=VECTOR('',#33501,1.);
#8933=VECTOR('',#33502,1.);
#8934=VECTOR('',#33503,1.);
#8935=VECTOR('',#33504,1.);
#8936=VECTOR('',#33507,1.);
#8937=VECTOR('',#33508,1.);
#8938=VECTOR('',#33511,1.);
#8939=VECTOR('',#33512,1.);
#8940=VECTOR('',#33515,1.);
#8941=VECTOR('',#33516,1.);
#8942=VECTOR('',#33519,1.);
#8943=VECTOR('',#33520,1.);
#8944=VECTOR('',#33523,1.);
#8945=VECTOR('',#33526,1.);
#8946=VECTOR('',#33535,0.0704);
#8947=VECTOR('',#33548,0.16);
#8948=VECTOR('',#33551,0.14375);
#10003=CIRCLE('',#27027,0.076925);
#10004=CIRCLE('',#27028,0.076925);
#10005=CIRCLE('',#27029,0.076925);
#10006=CIRCLE('',#27037,0.056925);
#10007=CIRCLE('',#27045,0.056925);
#10008=CIRCLE('',#27047,0.056925);
#10009=CIRCLE('',#27056,0.1275);
#10010=CIRCLE('',#27065,0.0608);
#10011=CIRCLE('',#27068,0.076925);
#10012=CIRCLE('',#27070,0.16);
#10013=CIRCLE('',#27072,0.16);
#12179=VERTEX_POINT('',#51280);
#12180=VERTEX_POINT('',#51281);
#12181=VERTEX_POINT('',#51283);
#12182=VERTEX_POINT('',#51300);
#12183=VERTEX_POINT('',#51302);
#12184=VERTEX_POINT('',#51305);
#12185=VERTEX_POINT('',#51321);
#12186=VERTEX_POINT('',#51322);
#12187=VERTEX_POINT('',#51369);
#12188=VERTEX_POINT('',#51370);
#12189=VERTEX_POINT('',#51417);
#12190=VERTEX_POINT('',#51418);
#12191=VERTEX_POINT('',#51471);
#12192=VERTEX_POINT('',#51472);
#12193=VERTEX_POINT('',#51519);
#12194=VERTEX_POINT('',#51520);
#12195=VERTEX_POINT('',#51567);
#12196=VERTEX_POINT('',#51568);
#12197=VERTEX_POINT('',#51621);
#12198=VERTEX_POINT('',#51622);
#12199=VERTEX_POINT('',#51624);
#12200=VERTEX_POINT('',#51631);
#12201=VERTEX_POINT('',#51639);
#12202=VERTEX_POINT('',#51640);
#12203=VERTEX_POINT('',#51664);
#12204=VERTEX_POINT('',#51665);
#12205=VERTEX_POINT('',#51689);
#12206=VERTEX_POINT('',#51690);
#12207=VERTEX_POINT('',#51713);
#12208=VERTEX_POINT('',#51714);
#12209=VERTEX_POINT('',#51738);
#12210=VERTEX_POINT('',#51739);
#12211=VERTEX_POINT('',#51763);
#12212=VERTEX_POINT('',#51764);
#12213=VERTEX_POINT('',#51787);
#12214=VERTEX_POINT('',#51788);
#12215=VERTEX_POINT('',#51790);
#12216=VERTEX_POINT('',#52020);
#12217=VERTEX_POINT('',#52086);
#12218=VERTEX_POINT('',#52395);
#12219=VERTEX_POINT('',#52459);
#12220=VERTEX_POINT('',#52460);
#12221=VERTEX_POINT('',#52462);
#12222=VERTEX_POINT('',#52464);
#12223=VERTEX_POINT('',#52468);
#12224=VERTEX_POINT('',#52469);
#12225=VERTEX_POINT('',#52471);
#12226=VERTEX_POINT('',#52473);
#12227=VERTEX_POINT('',#52477);
#12228=VERTEX_POINT('',#52478);
#12229=VERTEX_POINT('',#52480);
#12230=VERTEX_POINT('',#52482);
#12231=VERTEX_POINT('',#52486);
#12232=VERTEX_POINT('',#52488);
#12233=VERTEX_POINT('',#52495);
#12234=VERTEX_POINT('',#52497);
#12235=VERTEX_POINT('',#52501);
#12236=VERTEX_POINT('',#52503);
#12237=VERTEX_POINT('',#52505);
#12238=VERTEX_POINT('',#52508);
#12239=VERTEX_POINT('',#52510);
#12240=VERTEX_POINT('',#52514);
#12241=VERTEX_POINT('',#52518);
#12242=VERTEX_POINT('',#52522);
#12243=VERTEX_POINT('',#52526);
#12244=VERTEX_POINT('',#52535);
#12245=VERTEX_POINT('',#52542);
#12246=VERTEX_POINT('',#52545);
#15626=EDGE_CURVE('',#12179,#12180,#7073,.T.);
#15627=EDGE_CURVE('',#12179,#12181,#845,.T.);
#15628=EDGE_CURVE('',#12181,#12182,#10003,.T.);
#15629=EDGE_CURVE('',#12182,#12183,#7074,.T.);
#15630=EDGE_CURVE('',#12183,#12183,#10004,.T.);
#15631=EDGE_CURVE('',#12182,#12184,#10005,.T.);
#15632=EDGE_CURVE('',#12184,#12180,#846,.T.);
#15633=EDGE_CURVE('',#12185,#12186,#7075,.T.);
#15634=EDGE_CURVE('',#12185,#12179,#847,.T.);
#15635=EDGE_CURVE('',#12180,#12186,#848,.T.);
#15636=EDGE_CURVE('',#12187,#12188,#7076,.T.);
#15637=EDGE_CURVE('',#12187,#12185,#849,.T.);
#15638=EDGE_CURVE('',#12186,#12188,#850,.T.);
#15639=EDGE_CURVE('',#12189,#12190,#7077,.T.);
#15640=EDGE_CURVE('',#12189,#12187,#851,.T.);
#15641=EDGE_CURVE('',#12188,#12190,#852,.T.);
#15642=EDGE_CURVE('',#12191,#12192,#7078,.T.);
#15643=EDGE_CURVE('',#12191,#12189,#853,.T.);
#15644=EDGE_CURVE('',#12190,#12192,#854,.T.);
#15645=EDGE_CURVE('',#12193,#12194,#7079,.T.);
#15646=EDGE_CURVE('',#12193,#12191,#855,.T.);
#15647=EDGE_CURVE('',#12192,#12194,#856,.T.);
#15648=EDGE_CURVE('',#12195,#12196,#7080,.T.);
#15649=EDGE_CURVE('',#12195,#12193,#857,.T.);
#15650=EDGE_CURVE('',#12194,#12196,#858,.T.);
#15651=EDGE_CURVE('',#12197,#12198,#7081,.T.);
#15652=EDGE_CURVE('',#12197,#12199,#859,.T.);
#15653=EDGE_CURVE('',#12200,#12199,#10006,.T.);
#15654=EDGE_CURVE('',#12198,#12200,#860,.T.);
#15655=EDGE_CURVE('',#12201,#12202,#7082,.T.);
#15656=EDGE_CURVE('',#12201,#12197,#861,.T.);
#15657=EDGE_CURVE('',#12202,#12198,#862,.T.);
#15658=EDGE_CURVE('',#12203,#12204,#7083,.T.);
#15659=EDGE_CURVE('',#12203,#12201,#863,.T.);
#15660=EDGE_CURVE('',#12204,#12202,#864,.T.);
#15661=EDGE_CURVE('',#12205,#12206,#7084,.T.);
#15662=EDGE_CURVE('',#12205,#12203,#865,.T.);
#15663=EDGE_CURVE('',#12206,#12204,#866,.T.);
#15664=EDGE_CURVE('',#12207,#12208,#7085,.T.);
#15665=EDGE_CURVE('',#12207,#12205,#867,.T.);
#15666=EDGE_CURVE('',#12208,#12206,#868,.T.);
#15667=EDGE_CURVE('',#12209,#12210,#7086,.T.);
#15668=EDGE_CURVE('',#12209,#12207,#869,.T.);
#15669=EDGE_CURVE('',#12210,#12208,#870,.T.);
#15670=EDGE_CURVE('',#12211,#12212,#7087,.T.);
#15671=EDGE_CURVE('',#12211,#12209,#871,.T.);
#15672=EDGE_CURVE('',#12212,#12210,#872,.T.);
#15673=EDGE_CURVE('',#12213,#12214,#7088,.T.);
#15674=EDGE_CURVE('',#12215,#12213,#10007,.T.);
#15675=EDGE_CURVE('',#12215,#12211,#873,.T.);
#15676=EDGE_CURVE('',#12214,#12212,#874,.T.);
#15677=EDGE_CURVE('',#12216,#12200,#875,.T.);
#15678=EDGE_CURVE('',#12196,#12216,#876,.T.);
#15679=EDGE_CURVE('',#12217,#12184,#877,.T.);
#15680=EDGE_CURVE('',#12217,#12214,#878,.T.);
#15681=EDGE_CURVE('',#12181,#12215,#879,.T.);
#15682=EDGE_CURVE('',#12213,#12217,#10008,.T.);
#15683=EDGE_CURVE('',#12199,#12218,#880,.T.);
#15684=EDGE_CURVE('',#12218,#12195,#881,.T.);
#15685=EDGE_CURVE('',#12219,#12220,#7089,.T.);
#15686=EDGE_CURVE('',#12221,#12219,#7090,.T.);
#15687=EDGE_CURVE('',#12222,#12221,#7091,.T.);
#15688=EDGE_CURVE('',#12222,#12220,#7092,.T.);
#15689=EDGE_CURVE('',#12223,#12224,#7093,.T.);
#15690=EDGE_CURVE('',#12225,#12223,#7094,.T.);
#15691=EDGE_CURVE('',#12226,#12225,#7095,.T.);
#15692=EDGE_CURVE('',#12224,#12226,#7096,.T.);
#15693=EDGE_CURVE('',#12227,#12228,#7097,.T.);
#15694=EDGE_CURVE('',#12229,#12227,#7098,.T.);
#15695=EDGE_CURVE('',#12230,#12229,#7099,.T.);
#15696=EDGE_CURVE('',#12230,#12228,#7100,.T.);
#15697=EDGE_CURVE('',#12220,#12231,#7101,.T.);
#15698=EDGE_CURVE('',#12232,#12222,#7102,.T.);
#15699=EDGE_CURVE('',#12231,#12232,#7103,.T.);
#15700=EDGE_CURVE('',#12228,#12223,#7104,.T.);
#15701=EDGE_CURVE('',#12225,#12230,#7105,.T.);
#15702=EDGE_CURVE('',#12233,#12219,#7106,.T.);
#15703=EDGE_CURVE('',#12234,#12233,#7107,.T.);
#15704=EDGE_CURVE('',#12221,#12234,#7108,.T.);
#15705=EDGE_CURVE('',#12235,#12235,#10009,.T.);
#15706=EDGE_CURVE('',#12231,#12236,#7109,.T.);
#15707=EDGE_CURVE('',#12236,#12237,#7110,.T.);
#15708=EDGE_CURVE('',#12237,#12227,#7111,.T.);
#15709=EDGE_CURVE('',#12224,#12238,#7112,.T.);
#15710=EDGE_CURVE('',#12238,#12239,#7113,.T.);
#15711=EDGE_CURVE('',#12239,#12233,#7114,.T.);
#15712=EDGE_CURVE('',#12240,#12232,#7115,.T.);
#15713=EDGE_CURVE('',#12240,#12236,#7116,.T.);
#15714=EDGE_CURVE('',#12241,#12237,#7117,.T.);
#15715=EDGE_CURVE('',#12229,#12241,#7118,.T.);
#15716=EDGE_CURVE('',#12242,#12226,#7119,.T.);
#15717=EDGE_CURVE('',#12242,#12238,#7120,.T.);
#15718=EDGE_CURVE('',#12243,#12239,#7121,.T.);
#15719=EDGE_CURVE('',#12234,#12243,#7122,.T.);
#15720=EDGE_CURVE('',#12241,#12240,#7123,.T.);
#15721=EDGE_CURVE('',#12243,#12242,#7124,.T.);
#15722=EDGE_CURVE('',#12244,#12244,#10010,.T.);
#15723=EDGE_CURVE('',#12183,#12244,#7125,.T.);
#15724=EDGE_CURVE('',#12218,#12216,#10011,.T.);
#15725=EDGE_CURVE('',#12245,#12245,#10012,.T.);
#15726=EDGE_CURVE('',#12246,#12246,#10013,.T.);
#15727=EDGE_CURVE('',#12246,#12245,#7126,.T.);
#15728=EDGE_CURVE('',#12235,#12246,#7127,.T.);
#22436=ORIENTED_EDGE('',*,*,#15626,.F.);
#22437=ORIENTED_EDGE('',*,*,#15627,.T.);
#22438=ORIENTED_EDGE('',*,*,#15628,.T.);
#22439=ORIENTED_EDGE('',*,*,#15629,.T.);
#22440=ORIENTED_EDGE('',*,*,#15630,.T.);
#22441=ORIENTED_EDGE('',*,*,#15629,.F.);
#22442=ORIENTED_EDGE('',*,*,#15631,.T.);
#22443=ORIENTED_EDGE('',*,*,#15632,.T.);
#22444=ORIENTED_EDGE('',*,*,#15633,.F.);
#22445=ORIENTED_EDGE('',*,*,#15634,.T.);
#22446=ORIENTED_EDGE('',*,*,#15626,.T.);
#22447=ORIENTED_EDGE('',*,*,#15635,.T.);
#22448=ORIENTED_EDGE('',*,*,#15636,.F.);
#22449=ORIENTED_EDGE('',*,*,#15637,.T.);
#22450=ORIENTED_EDGE('',*,*,#15633,.T.);
#22451=ORIENTED_EDGE('',*,*,#15638,.T.);
#22452=ORIENTED_EDGE('',*,*,#15639,.F.);
#22453=ORIENTED_EDGE('',*,*,#15640,.T.);
#22454=ORIENTED_EDGE('',*,*,#15636,.T.);
#22455=ORIENTED_EDGE('',*,*,#15641,.T.);
#22456=ORIENTED_EDGE('',*,*,#15642,.F.);
#22457=ORIENTED_EDGE('',*,*,#15643,.T.);
#22458=ORIENTED_EDGE('',*,*,#15639,.T.);
#22459=ORIENTED_EDGE('',*,*,#15644,.T.);
#22460=ORIENTED_EDGE('',*,*,#15645,.F.);
#22461=ORIENTED_EDGE('',*,*,#15646,.T.);
#22462=ORIENTED_EDGE('',*,*,#15642,.T.);
#22463=ORIENTED_EDGE('',*,*,#15647,.T.);
#22464=ORIENTED_EDGE('',*,*,#15648,.F.);
#22465=ORIENTED_EDGE('',*,*,#15649,.T.);
#22466=ORIENTED_EDGE('',*,*,#15645,.T.);
#22467=ORIENTED_EDGE('',*,*,#15650,.T.);
#22468=ORIENTED_EDGE('',*,*,#15651,.F.);
#22469=ORIENTED_EDGE('',*,*,#15652,.T.);
#22470=ORIENTED_EDGE('',*,*,#15653,.F.);
#22471=ORIENTED_EDGE('',*,*,#15654,.F.);
#22472=ORIENTED_EDGE('',*,*,#15655,.F.);
#22473=ORIENTED_EDGE('',*,*,#15656,.T.);
#22474=ORIENTED_EDGE('',*,*,#15651,.T.);
#22475=ORIENTED_EDGE('',*,*,#15657,.F.);
#22476=ORIENTED_EDGE('',*,*,#15658,.F.);
#22477=ORIENTED_EDGE('',*,*,#15659,.T.);
#22478=ORIENTED_EDGE('',*,*,#15655,.T.);
#22479=ORIENTED_EDGE('',*,*,#15660,.F.);
#22480=ORIENTED_EDGE('',*,*,#15661,.F.);
#22481=ORIENTED_EDGE('',*,*,#15662,.T.);
#22482=ORIENTED_EDGE('',*,*,#15658,.T.);
#22483=ORIENTED_EDGE('',*,*,#15663,.F.);
#22484=ORIENTED_EDGE('',*,*,#15664,.F.);
#22485=ORIENTED_EDGE('',*,*,#15665,.T.);
#22486=ORIENTED_EDGE('',*,*,#15661,.T.);
#22487=ORIENTED_EDGE('',*,*,#15666,.F.);
#22488=ORIENTED_EDGE('',*,*,#15667,.F.);
#22489=ORIENTED_EDGE('',*,*,#15668,.T.);
#22490=ORIENTED_EDGE('',*,*,#15664,.T.);
#22491=ORIENTED_EDGE('',*,*,#15669,.F.);
#22492=ORIENTED_EDGE('',*,*,#15670,.F.);
#22493=ORIENTED_EDGE('',*,*,#15671,.T.);
#22494=ORIENTED_EDGE('',*,*,#15667,.T.);
#22495=ORIENTED_EDGE('',*,*,#15672,.F.);
#22496=ORIENTED_EDGE('',*,*,#15673,.F.);
#22497=ORIENTED_EDGE('',*,*,#15674,.F.);
#22498=ORIENTED_EDGE('',*,*,#15675,.T.);
#22499=ORIENTED_EDGE('',*,*,#15670,.T.);
#22500=ORIENTED_EDGE('',*,*,#15676,.F.);
#22501=ORIENTED_EDGE('',*,*,#15677,.F.);
#22502=ORIENTED_EDGE('',*,*,#15678,.F.);
#22503=ORIENTED_EDGE('',*,*,#15650,.F.);
#22504=ORIENTED_EDGE('',*,*,#15647,.F.);
#22505=ORIENTED_EDGE('',*,*,#15644,.F.);
#22506=ORIENTED_EDGE('',*,*,#15641,.F.);
#22507=ORIENTED_EDGE('',*,*,#15638,.F.);
#22508=ORIENTED_EDGE('',*,*,#15635,.F.);
#22509=ORIENTED_EDGE('',*,*,#15632,.F.);
#22510=ORIENTED_EDGE('',*,*,#15679,.F.);
#22511=ORIENTED_EDGE('',*,*,#15680,.T.);
#22512=ORIENTED_EDGE('',*,*,#15676,.T.);
#22513=ORIENTED_EDGE('',*,*,#15672,.T.);
#22514=ORIENTED_EDGE('',*,*,#15669,.T.);
#22515=ORIENTED_EDGE('',*,*,#15666,.T.);
#22516=ORIENTED_EDGE('',*,*,#15663,.T.);
#22517=ORIENTED_EDGE('',*,*,#15660,.T.);
#22518=ORIENTED_EDGE('',*,*,#15657,.T.);
#22519=ORIENTED_EDGE('',*,*,#15654,.T.);
#22520=ORIENTED_EDGE('',*,*,#15628,.F.);
#22521=ORIENTED_EDGE('',*,*,#15681,.T.);
#22522=ORIENTED_EDGE('',*,*,#15674,.T.);
#22523=ORIENTED_EDGE('',*,*,#15682,.T.);
#22524=ORIENTED_EDGE('',*,*,#15679,.T.);
#22525=ORIENTED_EDGE('',*,*,#15631,.F.);
#22526=ORIENTED_EDGE('',*,*,#15673,.T.);
#22527=ORIENTED_EDGE('',*,*,#15680,.F.);
#22528=ORIENTED_EDGE('',*,*,#15682,.F.);
#22529=ORIENTED_EDGE('',*,*,#15683,.F.);
#22530=ORIENTED_EDGE('',*,*,#15652,.F.);
#22531=ORIENTED_EDGE('',*,*,#15656,.F.);
#22532=ORIENTED_EDGE('',*,*,#15659,.F.);
#22533=ORIENTED_EDGE('',*,*,#15662,.F.);
#22534=ORIENTED_EDGE('',*,*,#15665,.F.);
#22535=ORIENTED_EDGE('',*,*,#15668,.F.);
#22536=ORIENTED_EDGE('',*,*,#15671,.F.);
#22537=ORIENTED_EDGE('',*,*,#15675,.F.);
#22538=ORIENTED_EDGE('',*,*,#15681,.F.);
#22539=ORIENTED_EDGE('',*,*,#15627,.F.);
#22540=ORIENTED_EDGE('',*,*,#15634,.F.);
#22541=ORIENTED_EDGE('',*,*,#15637,.F.);
#22542=ORIENTED_EDGE('',*,*,#15640,.F.);
#22543=ORIENTED_EDGE('',*,*,#15643,.F.);
#22544=ORIENTED_EDGE('',*,*,#15646,.F.);
#22545=ORIENTED_EDGE('',*,*,#15649,.F.);
#22546=ORIENTED_EDGE('',*,*,#15684,.F.);
#22547=ORIENTED_EDGE('',*,*,#15685,.F.);
#22548=ORIENTED_EDGE('',*,*,#15686,.F.);
#22549=ORIENTED_EDGE('',*,*,#15687,.F.);
#22550=ORIENTED_EDGE('',*,*,#15688,.T.);
#22551=ORIENTED_EDGE('',*,*,#15689,.F.);
#22552=ORIENTED_EDGE('',*,*,#15690,.F.);
#22553=ORIENTED_EDGE('',*,*,#15691,.F.);
#22554=ORIENTED_EDGE('',*,*,#15692,.F.);
#22555=ORIENTED_EDGE('',*,*,#15693,.F.);
#22556=ORIENTED_EDGE('',*,*,#15694,.F.);
#22557=ORIENTED_EDGE('',*,*,#15695,.F.);
#22558=ORIENTED_EDGE('',*,*,#15696,.T.);
#22559=ORIENTED_EDGE('',*,*,#15697,.F.);
#22560=ORIENTED_EDGE('',*,*,#15688,.F.);
#22561=ORIENTED_EDGE('',*,*,#15698,.F.);
#22562=ORIENTED_EDGE('',*,*,#15699,.F.);
#22563=ORIENTED_EDGE('',*,*,#15700,.F.);
#22564=ORIENTED_EDGE('',*,*,#15696,.F.);
#22565=ORIENTED_EDGE('',*,*,#15701,.F.);
#22566=ORIENTED_EDGE('',*,*,#15690,.T.);
#22567=ORIENTED_EDGE('',*,*,#15702,.F.);
#22568=ORIENTED_EDGE('',*,*,#15703,.F.);
#22569=ORIENTED_EDGE('',*,*,#15704,.F.);
#22570=ORIENTED_EDGE('',*,*,#15686,.T.);
#22571=ORIENTED_EDGE('',*,*,#15705,.T.);
#22572=ORIENTED_EDGE('',*,*,#15702,.T.);
#22573=ORIENTED_EDGE('',*,*,#15685,.T.);
#22574=ORIENTED_EDGE('',*,*,#15697,.T.);
#22575=ORIENTED_EDGE('',*,*,#15706,.T.);
#22576=ORIENTED_EDGE('',*,*,#15707,.T.);
#22577=ORIENTED_EDGE('',*,*,#15708,.T.);
#22578=ORIENTED_EDGE('',*,*,#15693,.T.);
#22579=ORIENTED_EDGE('',*,*,#15700,.T.);
#22580=ORIENTED_EDGE('',*,*,#15689,.T.);
#22581=ORIENTED_EDGE('',*,*,#15709,.T.);
#22582=ORIENTED_EDGE('',*,*,#15710,.T.);
#22583=ORIENTED_EDGE('',*,*,#15711,.T.);
#22584=ORIENTED_EDGE('',*,*,#15699,.T.);
#22585=ORIENTED_EDGE('',*,*,#15712,.F.);
#22586=ORIENTED_EDGE('',*,*,#15713,.T.);
#22587=ORIENTED_EDGE('',*,*,#15706,.F.);
#22588=ORIENTED_EDGE('',*,*,#15694,.T.);
#22589=ORIENTED_EDGE('',*,*,#15708,.F.);
#22590=ORIENTED_EDGE('',*,*,#15714,.F.);
#22591=ORIENTED_EDGE('',*,*,#15715,.F.);
#22592=ORIENTED_EDGE('',*,*,#15692,.T.);
#22593=ORIENTED_EDGE('',*,*,#15716,.F.);
#22594=ORIENTED_EDGE('',*,*,#15717,.T.);
#22595=ORIENTED_EDGE('',*,*,#15709,.F.);
#22596=ORIENTED_EDGE('',*,*,#15703,.T.);
#22597=ORIENTED_EDGE('',*,*,#15711,.F.);
#22598=ORIENTED_EDGE('',*,*,#15718,.F.);
#22599=ORIENTED_EDGE('',*,*,#15719,.F.);
#22600=ORIENTED_EDGE('',*,*,#15707,.F.);
#22601=ORIENTED_EDGE('',*,*,#15713,.F.);
#22602=ORIENTED_EDGE('',*,*,#15720,.F.);
#22603=ORIENTED_EDGE('',*,*,#15714,.T.);
#22604=ORIENTED_EDGE('',*,*,#15710,.F.);
#22605=ORIENTED_EDGE('',*,*,#15717,.F.);
#22606=ORIENTED_EDGE('',*,*,#15721,.F.);
#22607=ORIENTED_EDGE('',*,*,#15718,.T.);
#22608=ORIENTED_EDGE('',*,*,#15719,.T.);
#22609=ORIENTED_EDGE('',*,*,#15721,.T.);
#22610=ORIENTED_EDGE('',*,*,#15716,.T.);
#22611=ORIENTED_EDGE('',*,*,#15691,.T.);
#22612=ORIENTED_EDGE('',*,*,#15701,.T.);
#22613=ORIENTED_EDGE('',*,*,#15695,.T.);
#22614=ORIENTED_EDGE('',*,*,#15715,.T.);
#22615=ORIENTED_EDGE('',*,*,#15720,.T.);
#22616=ORIENTED_EDGE('',*,*,#15712,.T.);
#22617=ORIENTED_EDGE('',*,*,#15698,.T.);
#22618=ORIENTED_EDGE('',*,*,#15687,.T.);
#22619=ORIENTED_EDGE('',*,*,#15704,.T.);
#22620=ORIENTED_EDGE('',*,*,#15722,.F.);
#22621=ORIENTED_EDGE('',*,*,#15630,.F.);
#22622=ORIENTED_EDGE('',*,*,#15723,.T.);
#22623=ORIENTED_EDGE('',*,*,#15722,.T.);
#22624=ORIENTED_EDGE('',*,*,#15723,.F.);
#22625=ORIENTED_EDGE('',*,*,#15648,.T.);
#22626=ORIENTED_EDGE('',*,*,#15678,.T.);
#22627=ORIENTED_EDGE('',*,*,#15724,.F.);
#22628=ORIENTED_EDGE('',*,*,#15684,.T.);
#22629=ORIENTED_EDGE('',*,*,#15725,.F.);
#22630=ORIENTED_EDGE('',*,*,#15724,.T.);
#22631=ORIENTED_EDGE('',*,*,#15677,.T.);
#22632=ORIENTED_EDGE('',*,*,#15653,.T.);
#22633=ORIENTED_EDGE('',*,*,#15683,.T.);
#22634=ORIENTED_EDGE('',*,*,#15726,.F.);
#22635=ORIENTED_EDGE('',*,*,#15727,.T.);
#22636=ORIENTED_EDGE('',*,*,#15725,.T.);
#22637=ORIENTED_EDGE('',*,*,#15727,.F.);
#22638=ORIENTED_EDGE('',*,*,#15705,.F.);
#22639=ORIENTED_EDGE('',*,*,#15728,.T.);
#22640=ORIENTED_EDGE('',*,*,#15726,.T.);
#22641=ORIENTED_EDGE('',*,*,#15728,.F.);
#23161=CONICAL_SURFACE('',#27066,0.0704,0.785398163397448);
#23162=CONICAL_SURFACE('',#27073,0.14375,0.558599315343562);
#24433=ADVANCED_FACE('',(#3680),#2358,.T.);
#24434=ADVANCED_FACE('',(#3681),#2359,.T.);
#24435=ADVANCED_FACE('',(#3682),#2360,.T.);
#24436=ADVANCED_FACE('',(#3683),#2361,.T.);
#24437=ADVANCED_FACE('',(#3684),#2362,.T.);
#24438=ADVANCED_FACE('',(#3685),#2363,.T.);
#24439=ADVANCED_FACE('',(#3686),#2364,.T.);
#24440=ADVANCED_FACE('',(#3687),#2365,.T.);
#24441=ADVANCED_FACE('',(#3688),#2366,.T.);
#24442=ADVANCED_FACE('',(#3689),#2367,.T.);
#24443=ADVANCED_FACE('',(#3690),#2368,.T.);
#24444=ADVANCED_FACE('',(#3691),#2369,.T.);
#24445=ADVANCED_FACE('',(#3692),#2370,.T.);
#24446=ADVANCED_FACE('',(#3693),#2371,.T.);
#24447=ADVANCED_FACE('',(#3694),#2372,.T.);
#24448=ADVANCED_FACE('',(#3695),#480,.F.);
#24449=ADVANCED_FACE('',(#3696),#1918,.T.);
#24450=ADVANCED_FACE('',(#3697),#2373,.T.);
#24451=ADVANCED_FACE('',(#3698),#481,.F.);
#24452=ADVANCED_FACE('',(#3699),#1919,.F.);
#24453=ADVANCED_FACE('',(#3700),#1920,.F.);
#24454=ADVANCED_FACE('',(#3701),#1921,.F.);
#24455=ADVANCED_FACE('',(#3702),#1922,.F.);
#24456=ADVANCED_FACE('',(#3703),#1923,.F.);
#24457=ADVANCED_FACE('',(#3704),#1924,.F.);
#24458=ADVANCED_FACE('',(#3705,#1272),#1925,.T.);
#24459=ADVANCED_FACE('',(#3706),#1926,.F.);
#24460=ADVANCED_FACE('',(#3707),#1927,.F.);
#24461=ADVANCED_FACE('',(#3708),#1928,.F.);
#24462=ADVANCED_FACE('',(#3709),#1929,.F.);
#24463=ADVANCED_FACE('',(#3710),#1930,.F.);
#24464=ADVANCED_FACE('',(#3711),#1931,.F.);
#24465=ADVANCED_FACE('',(#3712),#1932,.T.);
#24466=ADVANCED_FACE('',(#3713),#1933,.T.);
#24467=ADVANCED_FACE('',(#3714),#23161,.T.);
#24468=ADVANCED_FACE('',(#3715),#2374,.T.);
#24469=ADVANCED_FACE('',(#3716,#1273),#1934,.T.);
#24470=ADVANCED_FACE('',(#3717),#2375,.T.);
#24471=ADVANCED_FACE('',(#3718),#23162,.T.);
#24547=CLOSED_SHELL('',(#24433,#24434,#24435,#24436,#24437,#24438,#24439,
#24440,#24441,#24442,#24443,#24444,#24445,#24446,#24447,#24448,#24449,#24450,
#24451,#24452,#24453,#24454,#24455,#24456,#24457,#24458,#24459,#24460,#24461,
#24462,#24463,#24464,#24465,#24466,#24467,#24468,#24469,#24470,#24471));
#27025=AXIS2_PLACEMENT_3D('',#51278,#33399,#33400);
#27026=AXIS2_PLACEMENT_3D('',#51279,#33401,#33402);
#27027=AXIS2_PLACEMENT_3D('',#51301,#33404,#33405);
#27028=AXIS2_PLACEMENT_3D('',#51304,#33407,#33408);
#27029=AXIS2_PLACEMENT_3D('',#51306,#33409,#33410);
#27030=AXIS2_PLACEMENT_3D('',#51320,#33411,#33412);
#27031=AXIS2_PLACEMENT_3D('',#51368,#33414,#33415);
#27032=AXIS2_PLACEMENT_3D('',#51416,#33417,#33418);
#27033=AXIS2_PLACEMENT_3D('',#51470,#33420,#33421);
#27034=AXIS2_PLACEMENT_3D('',#51518,#33423,#33424);
#27035=AXIS2_PLACEMENT_3D('',#51566,#33426,#33427);
#27036=AXIS2_PLACEMENT_3D('',#51620,#33429,#33430);
#27037=AXIS2_PLACEMENT_3D('',#51632,#33432,#33433);
#27038=AXIS2_PLACEMENT_3D('',#51638,#33434,#33435);
#27039=AXIS2_PLACEMENT_3D('',#51663,#33437,#33438);
#27040=AXIS2_PLACEMENT_3D('',#51688,#33440,#33441);
#27041=AXIS2_PLACEMENT_3D('',#51712,#33443,#33444);
#27042=AXIS2_PLACEMENT_3D('',#51737,#33446,#33447);
#27043=AXIS2_PLACEMENT_3D('',#51762,#33449,#33450);
#27044=AXIS2_PLACEMENT_3D('',#51786,#33452,#33453);
#27045=AXIS2_PLACEMENT_3D('',#51791,#33455,#33456);
#27046=AXIS2_PLACEMENT_3D('',#52138,#33457,#33458);
#27047=AXIS2_PLACEMENT_3D('',#52185,#33459,#33460);
#27048=AXIS2_PLACEMENT_3D('',#52186,#33461,#33462);
#27049=AXIS2_PLACEMENT_3D('',#52458,#33463,#33464);
#27050=AXIS2_PLACEMENT_3D('',#52467,#33469,#33470);
#27051=AXIS2_PLACEMENT_3D('',#52476,#33475,#33476);
#27052=AXIS2_PLACEMENT_3D('',#52485,#33481,#33482);
#27053=AXIS2_PLACEMENT_3D('',#52491,#33486,#33487);
#27054=AXIS2_PLACEMENT_3D('',#52494,#33490,#33491);
#27055=AXIS2_PLACEMENT_3D('',#52500,#33495,#33496);
#27056=AXIS2_PLACEMENT_3D('',#52502,#33497,#33498);
#27057=AXIS2_PLACEMENT_3D('',#52513,#33505,#33506);
#27058=AXIS2_PLACEMENT_3D('',#52517,#33509,#33510);
#27059=AXIS2_PLACEMENT_3D('',#52521,#33513,#33514);
#27060=AXIS2_PLACEMENT_3D('',#52525,#33517,#33518);
#27061=AXIS2_PLACEMENT_3D('',#52529,#33521,#33522);
#27062=AXIS2_PLACEMENT_3D('',#52531,#33524,#33525);
#27063=AXIS2_PLACEMENT_3D('',#52533,#33527,#33528);
#27064=AXIS2_PLACEMENT_3D('',#52534,#33529,#33530);
#27065=AXIS2_PLACEMENT_3D('',#52536,#33531,#33532);
#27066=AXIS2_PLACEMENT_3D('',#52537,#33533,#33534);
#27067=AXIS2_PLACEMENT_3D('',#52539,#33536,#33537);
#27068=AXIS2_PLACEMENT_3D('',#52540,#33538,#33539);
#27069=AXIS2_PLACEMENT_3D('',#52541,#33540,#33541);
#27070=AXIS2_PLACEMENT_3D('',#52543,#33542,#33543);
#27071=AXIS2_PLACEMENT_3D('',#52544,#33544,#33545);
#27072=AXIS2_PLACEMENT_3D('',#52546,#33546,#33547);
#27073=AXIS2_PLACEMENT_3D('',#52548,#33549,#33550);
#33399=DIRECTION('axis',(0.,0.,1.));
#33400=DIRECTION('refdir',(1.,0.,0.));
#33401=DIRECTION('center_axis',(0.,0.,1.));
#33402=DIRECTION('ref_axis',(1.,0.,0.));
#33403=DIRECTION('',(0.,0.,-1.));
#33404=DIRECTION('center_axis',(0.,0.,-1.));
#33405=DIRECTION('ref_axis',(1.,0.,0.));
#33406=DIRECTION('',(0.,0.,-1.));
#33407=DIRECTION('center_axis',(0.,0.,1.));
#33408=DIRECTION('ref_axis',(1.,0.,0.));
#33409=DIRECTION('center_axis',(0.,0.,-1.));
#33410=DIRECTION('ref_axis',(1.,0.,0.));
#33411=DIRECTION('center_axis',(0.,0.,1.));
#33412=DIRECTION('ref_axis',(1.,0.,0.));
#33413=DIRECTION('',(0.,0.,-1.));
#33414=DIRECTION('center_axis',(0.,0.,1.));
#33415=DIRECTION('ref_axis',(1.,0.,0.));
#33416=DIRECTION('',(0.,0.,-1.));
#33417=DIRECTION('center_axis',(0.,0.,1.));
#33418=DIRECTION('ref_axis',(1.,0.,0.));
#33419=DIRECTION('',(0.,0.,-1.));
#33420=DIRECTION('center_axis',(0.,0.,1.));
#33421=DIRECTION('ref_axis',(1.,0.,0.));
#33422=DIRECTION('',(0.,0.,-1.));
#33423=DIRECTION('center_axis',(0.,0.,1.));
#33424=DIRECTION('ref_axis',(1.,0.,0.));
#33425=DIRECTION('',(0.,0.,-1.));
#33426=DIRECTION('center_axis',(0.,0.,1.));
#33427=DIRECTION('ref_axis',(1.,0.,0.));
#33428=DIRECTION('',(0.,0.,-1.));
#33429=DIRECTION('center_axis',(0.,0.,1.));
#33430=DIRECTION('ref_axis',(-0.128707264998563,-0.991682630651858,0.));
#33431=DIRECTION('',(0.,0.,1.));
#33432=DIRECTION('center_axis',(0.,0.,1.));
#33433=DIRECTION('ref_axis',(1.,3.87383608070041E-14,0.));
#33434=DIRECTION('center_axis',(0.,0.,1.));
#33435=DIRECTION('ref_axis',(1.,3.87383608070041E-14,0.));
#33436=DIRECTION('',(0.,0.,1.));
#33437=DIRECTION('center_axis',(0.,0.,1.));
#33438=DIRECTION('ref_axis',(1.,3.87383608070041E-14,0.));
#33439=DIRECTION('',(0.,0.,1.));
#33440=DIRECTION('center_axis',(0.,0.,1.));
#33441=DIRECTION('ref_axis',(1.,3.87383608070041E-14,0.));
#33442=DIRECTION('',(0.,0.,1.));
#33443=DIRECTION('center_axis',(0.,0.,1.));
#33444=DIRECTION('ref_axis',(1.,3.87383608070041E-14,0.));
#33445=DIRECTION('',(0.,0.,1.));
#33446=DIRECTION('center_axis',(0.,0.,1.));
#33447=DIRECTION('ref_axis',(1.,3.87383608070041E-14,0.));
#33448=DIRECTION('',(0.,0.,1.));
#33449=DIRECTION('center_axis',(0.,0.,1.));
#33450=DIRECTION('ref_axis',(1.,3.87383608070041E-14,0.));
#33451=DIRECTION('',(0.,0.,1.));
#33452=DIRECTION('center_axis',(0.,0.,1.));
#33453=DIRECTION('ref_axis',(1.,3.87383608070041E-14,0.));
#33454=DIRECTION('',(0.,0.,1.));
#33455=DIRECTION('center_axis',(0.,0.,-1.));
#33456=DIRECTION('ref_axis',(1.,3.87383608070041E-14,0.));
#33457=DIRECTION('center_axis',(0.,0.,1.));
#33458=DIRECTION('ref_axis',(1.,0.,0.));
#33459=DIRECTION('center_axis',(0.,0.,-1.));
#33460=DIRECTION('ref_axis',(1.,3.87383608070041E-14,0.));
#33461=DIRECTION('center_axis',(0.,0.,1.));
#33462=DIRECTION('ref_axis',(1.,3.87383608070041E-14,0.));
#33463=DIRECTION('center_axis',(0.,-1.,0.));
#33464=DIRECTION('ref_axis',(1.,0.,0.));
#33465=DIRECTION('',(-1.,0.,0.));
#33466=DIRECTION('',(0.,0.,1.));
#33467=DIRECTION('',(1.,0.,0.));
#33468=DIRECTION('',(0.,0.,1.));
#33469=DIRECTION('center_axis',(1.,0.,0.));
#33470=DIRECTION('ref_axis',(0.,1.,0.));
#33471=DIRECTION('',(0.,-1.,0.));
#33472=DIRECTION('',(0.,0.,1.));
#33473=DIRECTION('',(0.,1.,0.));
#33474=DIRECTION('',(0.,0.,-1.));
#33475=DIRECTION('center_axis',(-1.,0.,0.));
#33476=DIRECTION('ref_axis',(0.,-1.,0.));
#33477=DIRECTION('',(0.,1.,0.));
#33478=DIRECTION('',(0.,0.,1.));
#33479=DIRECTION('',(0.,-1.,0.));
#33480=DIRECTION('',(0.,0.,1.));
#33481=DIRECTION('center_axis',(-1.,0.,0.));
#33482=DIRECTION('ref_axis',(0.,-1.,0.));
#33483=DIRECTION('',(0.,1.,0.));
#33484=DIRECTION('',(0.,-1.,0.));
#33485=DIRECTION('',(0.,0.,-1.));
#33486=DIRECTION('center_axis',(0.,1.,0.));
#33487=DIRECTION('ref_axis',(-1.,0.,0.));
#33488=DIRECTION('',(1.,0.,0.));
#33489=DIRECTION('',(-1.,0.,0.));
#33490=DIRECTION('center_axis',(1.,0.,0.));
#33491=DIRECTION('ref_axis',(0.,1.,0.));
#33492=DIRECTION('',(0.,-1.,0.));
#33493=DIRECTION('',(0.,0.,1.));
#33494=DIRECTION('',(0.,1.,0.));
#33495=DIRECTION('center_axis',(0.,0.,1.));
#33496=DIRECTION('ref_axis',(1.,0.,0.));
#33497=DIRECTION('center_axis',(0.,0.,1.));
#33498=DIRECTION('ref_axis',(1.,0.,0.));
#33499=DIRECTION('',(-1.,0.,0.));
#33500=DIRECTION('',(0.,1.,0.));
#33501=DIRECTION('',(1.,0.,0.));
#33502=DIRECTION('',(1.,0.,0.));
#33503=DIRECTION('',(0.,-1.,0.));
#33504=DIRECTION('',(-1.,0.,0.));
#33505=DIRECTION('center_axis',(0.,-1.,0.));
#33506=DIRECTION('ref_axis',(1.,0.,0.));
#33507=DIRECTION('',(1.,0.,0.));
#33508=DIRECTION('',(0.,0.,1.));
#33509=DIRECTION('center_axis',(0.,1.,0.));
#33510=DIRECTION('ref_axis',(-1.,0.,0.));
#33511=DIRECTION('',(0.,0.,1.));
#33512=DIRECTION('',(-1.,0.,0.));
#33513=DIRECTION('center_axis',(0.,1.,0.));
#33514=DIRECTION('ref_axis',(-1.,0.,0.));
#33515=DIRECTION('',(-1.,0.,0.));
#33516=DIRECTION('',(0.,0.,1.));
#33517=DIRECTION('center_axis',(0.,-1.,0.));
#33518=DIRECTION('ref_axis',(1.,0.,0.));
#33519=DIRECTION('',(0.,0.,1.));
#33520=DIRECTION('',(1.,0.,0.));
#33521=DIRECTION('center_axis',(-1.,0.,0.));
#33522=DIRECTION('ref_axis',(0.,-1.,0.));
#33523=DIRECTION('',(0.,-1.,0.));
#33524=DIRECTION('center_axis',(1.,0.,0.));
#33525=DIRECTION('ref_axis',(0.,1.,0.));
#33526=DIRECTION('',(0.,1.,0.));
#33527=DIRECTION('center_axis',(0.,0.,1.));
#33528=DIRECTION('ref_axis',(1.,0.,0.));
#33529=DIRECTION('center_axis',(0.,0.,-1.));
#33530=DIRECTION('ref_axis',(-1.,0.,0.));
#33531=DIRECTION('center_axis',(0.,0.,1.));
#33532=DIRECTION('ref_axis',(1.,0.,0.));
#33533=DIRECTION('center_axis',(0.,0.,1.));
#33534=DIRECTION('ref_axis',(1.,0.,0.));
#33535=DIRECTION('',(0.707106781186548,8.65956056235493E-17,-0.707106781186548));
#33536=DIRECTION('center_axis',(0.,0.,1.));
#33537=DIRECTION('ref_axis',(0.977648531888111,-0.210245922902257,0.));
#33538=DIRECTION('center_axis',(0.,0.,1.));
#33539=DIRECTION('ref_axis',(1.,0.,0.));
#33540=DIRECTION('center_axis',(0.,0.,-1.));
#33541=DIRECTION('ref_axis',(-1.,0.,0.));
#33542=DIRECTION('center_axis',(0.,0.,1.));
#33543=DIRECTION('ref_axis',(1.,0.,0.));
#33544=DIRECTION('center_axis',(0.,0.,1.));
#33545=DIRECTION('ref_axis',(1.,0.,0.));
#33546=DIRECTION('center_axis',(0.,0.,1.));
#33547=DIRECTION('ref_axis',(1.,0.,0.));
#33548=DIRECTION('',(0.,0.,-1.));
#33549=DIRECTION('center_axis',(0.,0.,-1.));
#33550=DIRECTION('ref_axis',(1.,0.,0.));
#33551=DIRECTION('',(-0.52999894000318,-6.49061505426384E-17,-0.847998304005088));
#51278=CARTESIAN_POINT('',(0.,0.,0.));
#51279=CARTESIAN_POINT('Origin',(0.,0.,-0.1404));
#51280=CARTESIAN_POINT('',(-0.0769107559639177,6.92925783995872E-5,-0.237610382907248));
#51281=CARTESIAN_POINT('',(-0.0768920912054452,6.13296515658117E-5,-0.242639617092752));
#51282=CARTESIAN_POINT('',(-0.076925,-9.42059550244101E-18,-0.1404));
#51283=CARTESIAN_POINT('',(0.0402078774433248,-0.0657264351496036,-0.2608));
#51284=CARTESIAN_POINT('Ctrl Pts',(-0.0769107559639177,6.92925783995872E-5,
-0.237610382907248));
#51285=CARTESIAN_POINT('Ctrl Pts',(-0.0769685167490698,0.00645933324294077,
-0.238073052764717));
#51286=CARTESIAN_POINT('Ctrl Pts',(-0.0762388107008733,0.0128364434973379,
-0.238535722622186));
#51287=CARTESIAN_POINT('Ctrl Pts',(-0.074670594402015,0.019000293291529,
-0.238998392479655));
#51288=CARTESIAN_POINT('Ctrl Pts',(-0.0683908780681301,0.0436826207615176,
-0.240851093196551));
#51289=CARTESIAN_POINT('Ctrl Pts',(-0.0486656758144597,0.0649453233519243,
-0.242703793913448));
#51290=CARTESIAN_POINT('Ctrl Pts',(-0.0245197323996812,0.0730479175280928,
-0.244556494630344));
#51291=CARTESIAN_POINT('Ctrl Pts',(-0.000373788984902864,0.0811505117042614,
-0.246409195347241));
#51292=CARTESIAN_POINT('Ctrl Pts',(0.0281928955909835,0.0760929974661918,
-0.248261896064137));
#51293=CARTESIAN_POINT('Ctrl Pts',(0.0480896295923508,0.0602015617017921,
-0.250114596781034));
#51294=CARTESIAN_POINT('Ctrl Pts',(0.0679863635937181,0.0443101259373923,
-0.25196729749793));
#51295=CARTESIAN_POINT('Ctrl Pts',(0.0792131470205665,0.0175847686466624,
-0.253819998214827));
#51296=CARTESIAN_POINT('Ctrl Pts',(0.0766524840100219,-0.00775899280922349,
-0.255672698931724));
#51297=CARTESIAN_POINT('Ctrl Pts',(0.0742902945731415,-0.0311383931267909,
-0.257381799287816));
#51298=CARTESIAN_POINT('Ctrl Pts',(0.0601951224862113,-0.0533420688434893,
-0.259090899643908));
#51299=CARTESIAN_POINT('Ctrl Pts',(0.0402078774433248,-0.0657264351496036,
-0.2608));
#51300=CARTESIAN_POINT('',(-0.076925,-9.42059550244101E-18,-0.2608));
#51301=CARTESIAN_POINT('Origin',(0.,0.,-0.2608));
#51302=CARTESIAN_POINT('',(-0.076925,-9.42059550244101E-18,-0.283875));
#51303=CARTESIAN_POINT('',(-0.076925,-9.42059550244101E-18,-0.1404));
#51304=CARTESIAN_POINT('Origin',(0.,0.,-0.283875));
#51305=CARTESIAN_POINT('',(0.0763850617480247,-0.00909823976109922,-0.2608));
#51306=CARTESIAN_POINT('Origin',(0.,0.,-0.2608));
#51307=CARTESIAN_POINT('Ctrl Pts',(0.0763850617480247,-0.00909823976109917,
-0.2608));
#51308=CARTESIAN_POINT('Ctrl Pts',(0.0794111003994919,0.0163071304328721,
-0.258947299283103));
#51309=CARTESIAN_POINT('Ctrl Pts',(0.0687417228149469,0.0431206585224096,
-0.257094598566207));
#51310=CARTESIAN_POINT('Ctrl Pts',(0.0491529311664505,0.0593298637717059,
-0.25524189784931));
#51311=CARTESIAN_POINT('Ctrl Pts',(0.029564139517954,0.0755390690210024,
-0.253389197132414));
#51312=CARTESIAN_POINT('Ctrl Pts',(0.00105593380550616,0.0811439514300577,
-0.251536496415517));
#51313=CARTESIAN_POINT('Ctrl Pts',(-0.0232378405355734,0.0734789981937897,
-0.249683795698621));
#51314=CARTESIAN_POINT('Ctrl Pts',(-0.0475316148766529,0.0658140449575217,
-0.247831094981724));
#51315=CARTESIAN_POINT('Ctrl Pts',(-0.0676109578463641,0.0448792560759306,
-0.245978394264828));
#51316=CARTESIAN_POINT('Ctrl Pts',(-0.0743200843287782,0.0203058807031412,
-0.244125693547931));
#51317=CARTESIAN_POINT('Ctrl Pts',(-0.0761139115435399,0.0137356677823074,
-0.243630334729538));
#51318=CARTESIAN_POINT('Ctrl Pts',(-0.0769519372805849,0.00690534191951837,
-0.243134975911145));
#51319=CARTESIAN_POINT('Ctrl Pts',(-0.0768920912054452,6.13296515658117E-5,
-0.242639617092752));
#51320=CARTESIAN_POINT('Origin',(0.,0.,-0.1404));
#51321=CARTESIAN_POINT('',(-0.0768031572226018,-1.95264706120274E-5,-0.202610382907248));
#51322=CARTESIAN_POINT('',(-0.076807157253071,-2.66424230989696E-5,-0.207639617092752));
#51323=CARTESIAN_POINT('',(-0.076925,-9.42059550244101E-18,-0.1404));
#51324=CARTESIAN_POINT('Ctrl Pts',(-0.0768031572226018,-1.95264706120274E-5,
-0.202610382907248));
#51325=CARTESIAN_POINT('Ctrl Pts',(-0.0767712748932385,0.0140231988469081,
-0.203623515130004));
#51326=CARTESIAN_POINT('Ctrl Pts',(-0.0730908430886916,0.0280814791033811,
-0.20463664735276));
#51327=CARTESIAN_POINT('Ctrl Pts',(-0.0658633246280591,0.0399862919354661,
-0.205649779575517));
#51328=CARTESIAN_POINT('Ctrl Pts',(-0.0526464627687379,0.0617564565527937,
-0.207502480292413));
#51329=CARTESIAN_POINT('Ctrl Pts',(-0.0275678150095582,0.0763252268972791,
-0.20935518100931));
#51330=CARTESIAN_POINT('Ctrl Pts',(-0.00210920191325928,0.0770223484917919,
-0.211207881726206));
#51331=CARTESIAN_POINT('Ctrl Pts',(0.0233494111830397,0.0777194700863047,
-0.213060582443103));
#51332=CARTESIAN_POINT('Ctrl Pts',(0.0491879896164579,0.0645449429308449,
-0.214913283159999));
#51333=CARTESIAN_POINT('Ctrl Pts',(0.0635764027686449,0.0435307922368906,
-0.216765983876896));
#51334=CARTESIAN_POINT('Ctrl Pts',(0.0779648159208319,0.0225166415429363,
-0.218618684593793));
#51335=CARTESIAN_POINT('Ctrl Pts',(0.0809030637917877,-0.00633713268951243,
-0.220471385310689));
#51336=CARTESIAN_POINT('Ctrl Pts',(0.0710463837048955,-0.0298206145785707,
-0.222324086027586));
#51337=CARTESIAN_POINT('Ctrl Pts',(0.0611897036180032,-0.0533040964676289,
-0.224176786744482));
#51338=CARTESIAN_POINT('Ctrl Pts',(0.038538095573263,-0.0714172860132967,
-0.226029487461379));
#51339=CARTESIAN_POINT('Ctrl Pts',(0.0134614150354561,-0.0758664580059033,
-0.227882188178275));
#51340=CARTESIAN_POINT('Ctrl Pts',(-0.0116152655023509,-0.0803156299985098,
-0.229734888895172));
#51341=CARTESIAN_POINT('Ctrl Pts',(-0.0391170185332245,-0.0711007844380552,
-0.231587589612069));
#51342=CARTESIAN_POINT('Ctrl Pts',(-0.0564507798416117,-0.0524423854830426,
-0.233440290328965));
#51343=CARTESIAN_POINT('Ctrl Pts',(-0.0694558285841694,-0.038443497212289,
-0.234830321188393));
#51344=CARTESIAN_POINT('Ctrl Pts',(-0.076737221266271,-0.0191287458788749,
-0.23622035204782));
#51345=CARTESIAN_POINT('Ctrl Pts',(-0.0769107559639177,6.92925783995872E-5,
-0.237610382907248));
#51346=CARTESIAN_POINT('Ctrl Pts',(-0.0768920912054452,6.13296515658117E-5,
-0.242639617092752));
#51347=CARTESIAN_POINT('Ctrl Pts',(-0.0767281058634428,-0.018692075476664,
-0.241282275194248));
#51348=CARTESIAN_POINT('Ctrl Pts',(-0.0698226746732161,-0.0375482415536338,
-0.239924933295745));
#51349=CARTESIAN_POINT('Ctrl Pts',(-0.0573676133020383,-0.0514373135287137,
-0.238567591397241));
#51350=CARTESIAN_POINT('Ctrl Pts',(-0.0403671057977673,-0.0703951705237914,
-0.236714890680345));
#51351=CARTESIAN_POINT('Ctrl Pts',(-0.0130271807941084,-0.0800989226499592,
-0.234862189963448));
#51352=CARTESIAN_POINT('Ctrl Pts',(0.0121250371607425,-0.0760933557253033,
-0.233009489246552));
#51353=CARTESIAN_POINT('Ctrl Pts',(0.0372772551155935,-0.0720877888006474,
-0.231156788529655));
#51354=CARTESIAN_POINT('Ctrl Pts',(0.0602417660216363,-0.0543729028251678,
-0.229304087812759));
#51355=CARTESIAN_POINT('Ctrl Pts',(0.070509742362668,-0.0310658065448274,
-0.227451387095862));
#51356=CARTESIAN_POINT('Ctrl Pts',(0.0807777187036996,-0.00775871026448711,
-0.225598686378965));
#51357=CARTESIAN_POINT('Ctrl Pts',(0.0783491604797202,0.0211405963207139,
-0.223745985662069));
#51358=CARTESIAN_POINT('Ctrl Pts',(0.0643332164174167,0.0424043769590272,
-0.221893284945172));
#51359=CARTESIAN_POINT('Ctrl Pts',(0.0503172723551132,0.0636681575973404,
-0.220040584228276));
#51360=CARTESIAN_POINT('Ctrl Pts',(0.0247139424544857,0.0772964122887658,
-0.218187883511379));
#51361=CARTESIAN_POINT('Ctrl Pts',(-0.000753157637863402,0.0770477869535545,
-0.216335182794483));
#51362=CARTESIAN_POINT('Ctrl Pts',(-0.0262202577302126,0.0767991616183431,
-0.214482482077586));
#51363=CARTESIAN_POINT('Ctrl Pts',(-0.0515511280142834,0.0626736562564949,
-0.21262978136069));
#51364=CARTESIAN_POINT('Ctrl Pts',(-0.0651490986593925,0.0411394228871772,
-0.210777080643793));
#51365=CARTESIAN_POINT('Ctrl Pts',(-0.072824944858416,0.0289836779109062,
-0.209731259460113));
#51366=CARTESIAN_POINT('Ctrl Pts',(-0.0767621851696059,0.014467193901455,
-0.208685438276432));
#51367=CARTESIAN_POINT('Ctrl Pts',(-0.076807157253071,-2.66424230989696E-5,
-0.207639617092752));
#51368=CARTESIAN_POINT('Origin',(0.,0.,-0.1404));
#51369=CARTESIAN_POINT('',(-0.0769835019150157,-6.04666404582025E-5,-0.167610382907248));
#51370=CARTESIAN_POINT('',(-0.0769958967773298,-5.59803197837138E-5,-0.172639617092752));
#51371=CARTESIAN_POINT('',(-0.076925,-9.42059550244101E-18,-0.1404));
#51372=CARTESIAN_POINT('Ctrl Pts',(-0.0769835019150157,-6.04666404582025E-5,
-0.167610382907248));
#51373=CARTESIAN_POINT('Ctrl Pts',(-0.0767976431805962,0.0214832714064119,
-0.169173977495292));
#51374=CARTESIAN_POINT('Ctrl Pts',(-0.0673441366562592,0.0431699129578856,
-0.170737572083335));
#51375=CARTESIAN_POINT('Ctrl Pts',(-0.0513089165162116,0.0574828694067931,
-0.172301166671379));
#51376=CARTESIAN_POINT('Ctrl Pts',(-0.0323088099180996,0.0744422685225056,
-0.174153867388276));
#51377=CARTESIAN_POINT('Ctrl Pts',(-0.00406808136104573,0.0810491302208425,
-0.176006568105172));
#51378=CARTESIAN_POINT('Ctrl Pts',(0.0204835983469324,0.0742785807479444,
-0.177859268822069));
#51379=CARTESIAN_POINT('Ctrl Pts',(0.0450352780549104,0.0675080312750463,
-0.179711969538965));
#51380=CARTESIAN_POINT('Ctrl Pts',(0.0658979089138128,0.0473600706309135,
-0.181564670255862));
#51381=CARTESIAN_POINT('Ctrl Pts',(0.073519784037494,0.0230592021375661,
-0.183417370972758));
#51382=CARTESIAN_POINT('Ctrl Pts',(0.0811416591611752,-0.00124166635578134,
-0.185270071689655));
#51383=CARTESIAN_POINT('Ctrl Pts',(0.0755227785496352,-0.0296954426983434,
-0.187122772406551));
#51384=CARTESIAN_POINT('Ctrl Pts',(0.0592356885267185,-0.0492749211921189,
-0.188975473123448));
#51385=CARTESIAN_POINT('Ctrl Pts',(0.0429485985038016,-0.0688543996858945,
-0.190828173840344));
#51386=CARTESIAN_POINT('Ctrl Pts',(0.015993299069508,-0.0795595803308835,
-0.192680874557241));
#51387=CARTESIAN_POINT('Ctrl Pts',(-0.00928907365455888,-0.0764892089010994,
-0.194533575274138));
#51388=CARTESIAN_POINT('Ctrl Pts',(-0.0345714463786257,-0.0734188374713153,
-0.196386275991034));
#51389=CARTESIAN_POINT('Ctrl Pts',(-0.0581808923924657,-0.0565729139667582,
-0.198238976707931));
#51390=CARTESIAN_POINT('Ctrl Pts',(-0.0693080774196544,-0.0336641727693947,
-0.200091677424827));
#51391=CARTESIAN_POINT('Ctrl Pts',(-0.074350464402127,-0.0232828644586075,
-0.200931245918967));
#51392=CARTESIAN_POINT('Ctrl Pts',(-0.0768295776627497,-0.0116565364122966,
-0.201770814413108));
#51393=CARTESIAN_POINT('Ctrl Pts',(-0.0768031572226018,-1.95264706120274E-5,
-0.202610382907248));
#51394=CARTESIAN_POINT('Ctrl Pts',(-0.076807157253071,-2.66424230989696E-5,
-0.207639617092752));
#51395=CARTESIAN_POINT('Ctrl Pts',(-0.0768418544405828,-0.0112090319850631,
-0.206832737559536));
#51396=CARTESIAN_POINT('Ctrl Pts',(-0.0745596622880536,-0.022377940415552,
-0.20602585802632));
#51397=CARTESIAN_POINT('Ctrl Pts',(-0.0698900106134843,-0.0324387856940936,
-0.205218978493103));
#51398=CARTESIAN_POINT('Ctrl Pts',(-0.0591678809163199,-0.0555397995292589,
-0.203366277776207));
#51399=CARTESIAN_POINT('Ctrl Pts',(-0.035858550515844,-0.0727988658228025,
-0.20151357705931));
#51400=CARTESIAN_POINT('Ctrl Pts',(-0.010634123895685,-0.0763138640352252,
-0.199660876342414));
#51401=CARTESIAN_POINT('Ctrl Pts',(0.0145903027244741,-0.079828862247648,
-0.197808175625517));
#51402=CARTESIAN_POINT('Ctrl Pts',(0.0417298255643163,-0.06959979237895,
-0.195955474908621));
#51403=CARTESIAN_POINT('Ctrl Pts',(0.0583590560517694,-0.05031005037711,
-0.194102774191724));
#51404=CARTESIAN_POINT('Ctrl Pts',(0.0749882865392224,-0.03102030837527,
-0.192250073474828));
#51405=CARTESIAN_POINT('Ctrl Pts',(0.0811072246742864,-0.00266989424028812,
-0.190397372757931));
#51406=CARTESIAN_POINT('Ctrl Pts',(0.073914330385439,0.0217613744332338,
-0.188544672041035));
#51407=CARTESIAN_POINT('Ctrl Pts',(0.0667214360965916,0.0461926431067557,
-0.186691971324138));
#51408=CARTESIAN_POINT('Ctrl Pts',(0.0462167093838328,0.0667047663188176,
-0.184839270607242));
#51409=CARTESIAN_POINT('Ctrl Pts',(0.0217880206488223,0.0739064790943958,
-0.182986569890345));
#51410=CARTESIAN_POINT('Ctrl Pts',(-0.00264066808618824,0.0811081918699739,
-0.181133869173448));
#51411=CARTESIAN_POINT('Ctrl Pts',(-0.0309933188434504,0.0749994942090683,
-0.179281168456552));
#51412=CARTESIAN_POINT('Ctrl Pts',(-0.0502890320799736,0.0583771995879325,
-0.177428467739655));
#51413=CARTESIAN_POINT('Ctrl Pts',(-0.066914183311445,0.0440554609456219,
-0.175832184190688));
#51414=CARTESIAN_POINT('Ctrl Pts',(-0.0768159042207944,0.0219289387950761,
-0.17423590064172));
#51415=CARTESIAN_POINT('Ctrl Pts',(-0.0769958967773298,-5.59803197837138E-5,
-0.172639617092752));
#51416=CARTESIAN_POINT('Origin',(0.,0.,-0.1404));
#51417=CARTESIAN_POINT('',(-0.0769940708635155,5.67089128405991E-5,-0.132610382907248));
#51418=CARTESIAN_POINT('',(-0.0769815700716422,6.10755343289724E-5,-0.137639617092752));
#51419=CARTESIAN_POINT('',(-0.076925,-9.42059550244101E-18,-0.1404));
#51420=CARTESIAN_POINT('Ctrl Pts',(-0.0769940708635155,5.67089128405991E-5,
-0.132610382907248));
#51421=CARTESIAN_POINT('Ctrl Pts',(-0.0770238103898011,0.00365647805096637,
-0.132871739143682));
#51422=CARTESIAN_POINT('Ctrl Pts',(-0.0767931990646562,0.0072524177611427,
-0.133133095380117));
#51423=CARTESIAN_POINT('Ctrl Pts',(-0.0762891701184668,0.0108096161986601,
-0.133394451616551));
#51424=CARTESIAN_POINT('Ctrl Pts',(-0.0727162123705239,0.0360258658096909,
-0.135247152333448));
#51425=CARTESIAN_POINT('Ctrl Pts',(-0.0554037427351246,0.0592953273015094,
-0.137099853050345));
#51426=CARTESIAN_POINT('Ctrl Pts',(-0.0322780646014716,0.0699643611084238,
-0.138952553767241));
#51427=CARTESIAN_POINT('Ctrl Pts',(-0.00915238646781869,0.0806333949153382,
-0.140805254484138));
#51428=CARTESIAN_POINT('Ctrl Pts',(0.0197865001640878,0.0787020010373485,
-0.142657955201034));
#51429=CARTESIAN_POINT('Ctrl Pts',(0.0412892785043032,0.065054444597746,
-0.144510655917931));
#51430=CARTESIAN_POINT('Ctrl Pts',(0.0627920568445187,0.0514068881581433,
-0.146363356634827));
#51431=CARTESIAN_POINT('Ctrl Pts',(0.0768587268930429,0.0260431691569276,
-0.148216057351724));
#51432=CARTESIAN_POINT('Ctrl Pts',(0.0770490349640221,0.000575757562533098,
-0.15006875806862));
#51433=CARTESIAN_POINT('Ctrl Pts',(0.0772393430350013,-0.0248916540318611,
-0.151921458785517));
#51434=CARTESIAN_POINT('Ctrl Pts',(0.0635532891284355,-0.0504627582194342,
-0.153774159502413));
#51435=CARTESIAN_POINT('Ctrl Pts',(0.0422568665736587,-0.0644301365446651,
-0.15562686021931));
#51436=CARTESIAN_POINT('Ctrl Pts',(0.0209604440188819,-0.078397514869896,
-0.157479560936207));
#51437=CARTESIAN_POINT('Ctrl Pts',(-0.00794634718410591,-0.0807611673327848,
-0.159332261653103));
#51438=CARTESIAN_POINT('Ctrl Pts',(-0.0312288851198616,-0.0704389240607994,
-0.16118496237));
#51439=CARTESIAN_POINT('Ctrl Pts',(-0.0545114230556172,-0.0601166807888141,
-0.163037663086896));
#51440=CARTESIAN_POINT('Ctrl Pts',(-0.0721697077241406,-0.0371085417819546,
-0.164890363803793));
#51441=CARTESIAN_POINT('Ctrl Pts',(-0.0761191077388172,-0.0119485040119809,
-0.166743064520689));
#51442=CARTESIAN_POINT('Ctrl Pts',(-0.0767353949454457,-0.00802238628819954,
-0.167032170649542));
#51443=CARTESIAN_POINT('Ctrl Pts',(-0.0770178668965988,-0.00404386921512726,
-0.167321276778395));
#51444=CARTESIAN_POINT('Ctrl Pts',(-0.0769835019150157,-6.04666404582025E-5,
-0.167610382907248));
#51445=CARTESIAN_POINT('Ctrl Pts',(-0.0769958967773298,-5.59803197837138E-5,
-0.172639617092752));
#51446=CARTESIAN_POINT('Ctrl Pts',(-0.0770248096741801,-0.0035875024608357,
-0.172383199924823));
#51447=CARTESIAN_POINT('Ctrl Pts',(-0.0768028705500182,-0.00711537078577657,
-0.172126782756894));
#51448=CARTESIAN_POINT('Ctrl Pts',(-0.0763176518415591,-0.0106066485349346,
-0.171870365588966));
#51449=CARTESIAN_POINT('Ctrl Pts',(-0.0728117826508375,-0.0358323104552998,
-0.170017664872069));
#51450=CARTESIAN_POINT('Ctrl Pts',(-0.0555612685536102,-0.0591477427146643,
-0.168164964155173));
#51451=CARTESIAN_POINT('Ctrl Pts',(-0.0324640518946935,-0.0698782528471297,
-0.166312263438276));
#51452=CARTESIAN_POINT('Ctrl Pts',(-0.00936683523577665,-0.0806087629795951,
-0.16445956272138));
#51453=CARTESIAN_POINT('Ctrl Pts',(0.0195770839848297,-0.0787543509851614,
-0.162606862004483));
#51454=CARTESIAN_POINT('Ctrl Pts',(0.0411160872190435,-0.0651640398372977,
-0.160754161287586));
#51455=CARTESIAN_POINT('Ctrl Pts',(0.0626550904532573,-0.0515737286894341,
-0.15890146057069));
#51456=CARTESIAN_POINT('Ctrl Pts',(0.0767891777010786,-0.0262475183881405,
-0.157048759853793));
#51457=CARTESIAN_POINT('Ctrl Pts',(0.0770472279776439,-0.000780704307396157,
-0.155196059136897));
#51458=CARTESIAN_POINT('Ctrl Pts',(0.0773052782542091,0.0246861097733482,
-0.15334335842));
#51459=CARTESIAN_POINT('Ctrl Pts',(0.0636872915595182,0.0502935276335436,
-0.151490657703104));
#51460=CARTESIAN_POINT('Ctrl Pts',(0.0424280979279968,0.0643175040091825,
-0.149637956986207));
#51461=CARTESIAN_POINT('Ctrl Pts',(0.0211689042964752,0.0783414803848215,
-0.14778525626931));
#51462=CARTESIAN_POINT('Ctrl Pts',(-0.00773149627187655,0.080782015275904,
-0.145932555552414));
#51463=CARTESIAN_POINT('Ctrl Pts',(-0.0310414076692225,0.0705217399440169,
-0.144079854835518));
#51464=CARTESIAN_POINT('Ctrl Pts',(-0.0543513190665685,0.0602614646121299,
-0.142227154118621));
#51465=CARTESIAN_POINT('Ctrl Pts',(-0.0720707412929083,0.0373003790572733,
-0.140374453401724));
#51466=CARTESIAN_POINT('Ctrl Pts',(-0.0760870524860517,0.0121509364549594,
-0.138521752684828));
#51467=CARTESIAN_POINT('Ctrl Pts',(-0.0767244878832914,0.00815942679232915,
-0.138227707487469));
#51468=CARTESIAN_POINT('Ctrl Pts',(-0.0770167502794287,0.0041127937516773,
-0.137933662290111));
#51469=CARTESIAN_POINT('Ctrl Pts',(-0.0769815700716422,6.10755343289724E-5,
-0.137639617092752));
#51470=CARTESIAN_POINT('Origin',(0.,0.,-0.1404));
#51471=CARTESIAN_POINT('',(-0.0768065340016711,2.55117277794884E-5,-0.097610382907248));
#51472=CARTESIAN_POINT('',(-0.0768026632099214,1.84305570967413E-5,-0.102639617092752));
#51473=CARTESIAN_POINT('',(-0.076925,-9.42059550244101E-18,-0.1404));
#51474=CARTESIAN_POINT('Ctrl Pts',(-0.0768065340016711,2.55117277794884E-5,
-0.097610382907248));
#51475=CARTESIAN_POINT('Ctrl Pts',(-0.0768400025741158,0.0112766656092284,
-0.0984222015089698));
#51476=CARTESIAN_POINT('Ctrl Pts',(-0.0745285853311949,0.0225147292215057,
-0.0992340201106917));
#51477=CARTESIAN_POINT('Ctrl Pts',(-0.0698034168638814,0.0326246560661289,
-0.100045838712414));
#51478=CARTESIAN_POINT('Ctrl Pts',(-0.059019821873226,0.0556971363875672,
-0.10189853942931));
#51479=CARTESIAN_POINT('Ctrl Pts',(-0.0356647862302525,0.0728939886496841,
-0.103751240146207));
#51480=CARTESIAN_POINT('Ctrl Pts',(-0.0104311268550819,0.0763418424169287,
-0.105603940863103));
#51481=CARTESIAN_POINT('Ctrl Pts',(0.0148025325200884,0.0797896961841732,
-0.10745664158));
#51482=CARTESIAN_POINT('Ctrl Pts',(0.0419148156274558,0.0694885514565458,
-0.109309342296896));
#51483=CARTESIAN_POINT('Ctrl Pts',(0.0584926929014032,0.0501546624534022,
-0.111162043013793));
#51484=CARTESIAN_POINT('Ctrl Pts',(0.0750705701753508,0.0308207734502583,
-0.113014743730689));
#51485=CARTESIAN_POINT('Ctrl Pts',(0.0811140416158781,0.00245414017159807,
-0.114867444447586));
#51486=CARTESIAN_POINT('Ctrl Pts',(0.0738561779002024,-0.0219579200691195,
-0.116720145164483));
#51487=CARTESIAN_POINT('Ctrl Pts',(0.0665983141845268,-0.0463699803098367,
-0.118572845881379));
#51488=CARTESIAN_POINT('Ctrl Pts',(0.0460391153126481,-0.0668274675126116,
-0.120425546598276));
#51489=CARTESIAN_POINT('Ctrl Pts',(0.021591359872017,-0.0739641701402441,
-0.122278247315172));
#51490=CARTESIAN_POINT('Ctrl Pts',(-0.00285639556861437,-0.0811008727678766,
-0.124130948032069));
#51491=CARTESIAN_POINT('Ctrl Pts',(-0.0311927075779979,-0.074916790820367,
-0.125983648748965));
#51492=CARTESIAN_POINT('Ctrl Pts',(-0.0504441406524469,-0.0582432309814905,
-0.127836349465862));
#51493=CARTESIAN_POINT('Ctrl Pts',(-0.0669798182633061,-0.0439217719475156,
-0.129427693946324));
#51494=CARTESIAN_POINT('Ctrl Pts',(-0.0768129929919797,-0.0218615465190703,
-0.131019038426786));
#51495=CARTESIAN_POINT('Ctrl Pts',(-0.0769940708635155,5.67089128405991E-5,
-0.132610382907248));
#51496=CARTESIAN_POINT('Ctrl Pts',(-0.0769815700716422,6.10755343289724E-5,
-0.137639617092752));
#51497=CARTESIAN_POINT('Ctrl Pts',(-0.0767950891308295,-0.0214160069679987,
-0.136080961573214));
#51498=CARTESIAN_POINT('Ctrl Pts',(-0.0674081959306611,-0.0430359716776464,
-0.134522306053676));
#51499=CARTESIAN_POINT('Ctrl Pts',(-0.0514616363966927,-0.0573461837245798,
-0.132963650534138));
#51500=CARTESIAN_POINT('Ctrl Pts',(-0.0325067089542431,-0.0743560616520345,
-0.131110949817242));
#51501=CARTESIAN_POINT('Ctrl Pts',(-0.00428365390939655,-0.0810380178571733,
-0.129258249100345));
#51502=CARTESIAN_POINT('Ctrl Pts',(0.0202859467151432,-0.0743328001131744,
-0.127405548383449));
#51503=CARTESIAN_POINT('Ctrl Pts',(0.0448555473396833,-0.0676275823691754,
-0.125552847666552));
#51504=CARTESIAN_POINT('Ctrl Pts',(0.0657716935439163,-0.0475351906760383,
-0.123700146949655));
#51505=CARTESIAN_POINT('Ctrl Pts',(0.073458182507608,-0.0232546818828749,
-0.121847446232759));
#51506=CARTESIAN_POINT('Ctrl Pts',(0.0811446714712997,0.00102582691028839,
-0.119994745515862));
#51507=CARTESIAN_POINT('Ctrl Pts',(0.0756015031944501,0.0294944528034778,
-0.118142044798966));
#51508=CARTESIAN_POINT('Ctrl Pts',(0.0593665497202859,0.0491171821535752,
-0.116289344082069));
#51509=CARTESIAN_POINT('Ctrl Pts',(0.0431315962461219,0.0687399115036725,
-0.114436643365173));
#51510=CARTESIAN_POINT('Ctrl Pts',(0.016204857574643,0.0795167443106779,
-0.112583942648276));
#51511=CARTESIAN_POINT('Ctrl Pts',(-0.00908558679109352,0.076513638819554,
-0.11073124193138));
#51512=CARTESIAN_POINT('Ctrl Pts',(-0.0343760311568303,0.07351053332843,
-0.108878541214483));
#51513=CARTESIAN_POINT('Ctrl Pts',(-0.058030181216825,0.0567274895391765,
-0.107025840497587));
#51514=CARTESIAN_POINT('Ctrl Pts',(-0.0692182726444968,0.0338484198586954,
-0.10517313978069));
#51515=CARTESIAN_POINT('Ctrl Pts',(-0.0743180859797396,0.0234195647310118,
-0.104328632218044));
#51516=CARTESIAN_POINT('Ctrl Pts',(-0.0768277445635456,0.0117240983276437,
-0.103484124655398));
#51517=CARTESIAN_POINT('Ctrl Pts',(-0.0768026632099214,1.84305570967413E-5,
-0.102639617092752));
#51518=CARTESIAN_POINT('Origin',(0.,0.,-0.1404));
#51519=CARTESIAN_POINT('',(-0.0769006083194561,-6.96495813230711E-5,-0.062610382907248));
#51520=CARTESIAN_POINT('',(-0.0769139474189681,-7.03763467951925E-5,-0.0676396170927522));
#51521=CARTESIAN_POINT('',(-0.076925,-9.42059550244101E-18,-0.1404));
#51522=CARTESIAN_POINT('Ctrl Pts',(-0.0769006083194561,-6.96495813230711E-5,
-0.062610382907248));
#51523=CARTESIAN_POINT('Ctrl Pts',(-0.0767339796246602,0.0187523617936226,
-0.0639726638742573));
#51524=CARTESIAN_POINT('Ctrl Pts',(-0.069766977212752,0.0376847076479654,
-0.0653349448412665));
#51525=CARTESIAN_POINT('Ctrl Pts',(-0.0572276721267053,0.0515933582621614,
-0.0666972258082757));
#51526=CARTESIAN_POINT('Ctrl Pts',(-0.0401742300799402,0.0705091088217225,
-0.0685499265251723));
#51527=CARTESIAN_POINT('Ctrl Pts',(-0.0128142725637799,0.0801330466902033,
-0.0704026272420688));
#51528=CARTESIAN_POINT('Ctrl Pts',(0.0123258579767334,0.0760589202460425,
-0.0722553279589653));
#51529=CARTESIAN_POINT('Ctrl Pts',(0.037465988517247,0.0719847938018817,
-0.0741080286758619));
#51530=CARTESIAN_POINT('Ctrl Pts',(0.0603862920821135,0.0542126030450788,
-0.0759607293927584));
#51531=CARTESIAN_POINT('Ctrl Pts',(0.0705929441493049,0.0308791548460925,
-0.0778134301096549));
#51532=CARTESIAN_POINT('Ctrl Pts',(0.0807995962164963,0.0075457066471062,
-0.0796661308265515));
#51533=CARTESIAN_POINT('Ctrl Pts',(0.0782925967860125,-0.0213489989940634,
-0.0815188315434481));
#51534=CARTESIAN_POINT('Ctrl Pts',(0.064219767501604,-0.0425758865528817,
-0.0833715322603447));
#51535=CARTESIAN_POINT('Ctrl Pts',(0.0501469382171956,-0.0638027741116999,
-0.0852242329772412));
#51536=CARTESIAN_POINT('Ctrl Pts',(0.0245082790788626,-0.0773618435881669,
-0.0870769336941378));
#51537=CARTESIAN_POINT('Ctrl Pts',(-0.000957873902260806,-0.0770452329850995,
-0.0889296344110343));
#51538=CARTESIAN_POINT('Ctrl Pts',(-0.0264240268833843,-0.0767286223820321,
-0.0907823351279308));
#51539=CARTESIAN_POINT('Ctrl Pts',(-0.0517176737072984,-0.0625363316994301,
-0.0926350358448274));
#51540=CARTESIAN_POINT('Ctrl Pts',(-0.0652584199500865,-0.0409661321677492,
-0.0944877365617239));
#51541=CARTESIAN_POINT('Ctrl Pts',(-0.0728658659135372,-0.0288475882990529,
-0.0955286186768986));
#51542=CARTESIAN_POINT('Ctrl Pts',(-0.0767636219048009,-0.0144002784985585,
-0.0965695007920733));
#51543=CARTESIAN_POINT('Ctrl Pts',(-0.0768065340016711,2.55117277794884E-5,
-0.097610382907248));
#51544=CARTESIAN_POINT('Ctrl Pts',(-0.0768026632099214,1.84305570967413E-5,
-0.102639617092752));
#51545=CARTESIAN_POINT('Ctrl Pts',(-0.0767727204952061,-0.013956073206045,
-0.101631423938501));
#51546=CARTESIAN_POINT('Ctrl Pts',(-0.0731302282531401,-0.0279451161113039,
-0.100623230784251));
#51547=CARTESIAN_POINT('Ctrl Pts',(-0.0659694723256156,-0.0398109725683601,
-0.0996150376300002));
#51548=CARTESIAN_POINT('Ctrl Pts',(-0.0528105477837138,-0.0616161997432264,
-0.0977623369131037));
#51549=CARTESIAN_POINT('Ctrl Pts',(-0.027770665904561,-0.0762515585212508,
-0.0959096361962073));
#51550=CARTESIAN_POINT('Ctrl Pts',(-0.00231403248726689,-0.0770164274158603,
-0.0940569354793108));
#51551=CARTESIAN_POINT('Ctrl Pts',(0.0231426009300273,-0.0777812963104697,
-0.0922042347624142));
#51552=CARTESIAN_POINT('Ctrl Pts',(0.0490159858854629,-0.0646756753216641,
-0.0903515340455175));
#51553=CARTESIAN_POINT('Ctrl Pts',(0.0634603097011373,-0.0436998147451068,
-0.0884988333286209));
#51554=CARTESIAN_POINT('Ctrl Pts',(0.0779046335168115,-0.0227239541685498,
-0.0866461326117244));
#51555=CARTESIAN_POINT('Ctrl Pts',(0.0809198961927247,0.00612214599575843,
-0.084793431894828));
#51556=CARTESIAN_POINT('Ctrl Pts',(0.0711255935060718,0.0296316525829691,
-0.0829407311779315));
#51557=CARTESIAN_POINT('Ctrl Pts',(0.0613312908194188,0.05314115917018,
-0.0810880304610349));
#51558=CARTESIAN_POINT('Ctrl Pts',(0.0387274227701992,0.0713140721802931,
-0.0792353297441383));
#51559=CARTESIAN_POINT('Ctrl Pts',(0.0136629006290876,0.0758301399323035,
-0.0773826290272417));
#51560=CARTESIAN_POINT('Ctrl Pts',(-0.0114016215120237,0.0803462076843139,
-0.0755299283103452));
#51561=CARTESIAN_POINT('Ctrl Pts',(-0.038926797745027,0.0712054301782222,
-0.0736772275934487));
#51562=CARTESIAN_POINT('Ctrl Pts',(-0.0563105718570226,0.0525928101208236,
-0.0718245268765522));
#51563=CARTESIAN_POINT('Ctrl Pts',(-0.0693994868118571,0.0385786495911013,
-0.0704295569486189));
#51564=CARTESIAN_POINT('Ctrl Pts',(-0.0767390728503088,0.0191947445603847,
-0.0690345870206855));
#51565=CARTESIAN_POINT('Ctrl Pts',(-0.0769139474189681,-7.03763467951925E-5,
-0.0676396170927522));
#51566=CARTESIAN_POINT('Origin',(0.,0.,-0.1404));
#51567=CARTESIAN_POINT('',(-0.0770493699172285,1.64405594954022E-5,-0.027610382907248));
#51568=CARTESIAN_POINT('',(-0.0770428135801558,2.35063928346054E-5,-0.0326396170927521));
#51569=CARTESIAN_POINT('',(-0.076925,-9.42059550244101E-18,-0.1404));
#51570=CARTESIAN_POINT('Ctrl Pts',(-0.0770493699172285,1.64405594954022E-5,
-0.027610382907248));
#51571=CARTESIAN_POINT('Ctrl Pts',(-0.0770516866976547,0.000841965750576208,
-0.0276704255226481));
#51572=CARTESIAN_POINT('Ctrl Pts',(-0.0770396341883357,0.00166742001064634,
-0.0277304681380481));
#51573=CARTESIAN_POINT('Ctrl Pts',(-0.0770130084973636,0.00249239931151181,
-0.0277905107534482));
#51574=CARTESIAN_POINT('Ctrl Pts',(-0.076191434746402,0.0279483147801234,
-0.0296432114703447));
#51575=CARTESIAN_POINT('Ctrl Pts',(-0.0614944545164623,0.0529520124570084,
-0.0314959121872412));
#51576=CARTESIAN_POINT('Ctrl Pts',(-0.0396580599576723,0.0660601778222555,
-0.0333486129041378));
#51577=CARTESIAN_POINT('Ctrl Pts',(-0.0178216653988821,0.0791683431875028,
-0.0352013136210344));
#51578=CARTESIAN_POINT('Ctrl Pts',(0.0111541434887584,0.0803809762411121,
-0.037054014337931));
#51579=CARTESIAN_POINT('Ctrl Pts',(0.0340069177013224,0.0691406095455749,
-0.0389067150548276));
#51580=CARTESIAN_POINT('Ctrl Pts',(0.0568596919138859,0.057900242850038,
-0.0407594157717241));
#51581=CARTESIAN_POINT('Ctrl Pts',(0.0735894314513733,0.0342068764053553,
-0.0426121164886206));
#51582=CARTESIAN_POINT('Ctrl Pts',(0.0765346405079689,0.00890943025306635,
-0.0444648172055171));
#51583=CARTESIAN_POINT('Ctrl Pts',(0.0794798495645645,-0.0163880158992229,
-0.0463175179224137));
#51584=CARTESIAN_POINT('Ctrl Pts',(0.068640528140268,-0.0432895417591185,
-0.0481702186393103));
#51585=CARTESIAN_POINT('Ctrl Pts',(0.048980375614107,-0.0594792442461057,
-0.0500229193562068));
#51586=CARTESIAN_POINT('Ctrl Pts',(0.0293202230879464,-0.0756689467330926,
-0.0518756200731034));
#51587=CARTESIAN_POINT('Ctrl Pts',(0.000839239459921554,-0.0811468258471716,
-0.0537283207899999));
#51588=CARTESIAN_POINT('Ctrl Pts',(-0.0234234562141086,-0.07340456771045,
-0.0555810215068964));
#51589=CARTESIAN_POINT('Ctrl Pts',(-0.0476861518881389,-0.0656623095737284,
-0.057433722223793));
#51590=CARTESIAN_POINT('Ctrl Pts',(-0.0677305596081746,-0.044699914186206,
-0.0592864229406895));
#51591=CARTESIAN_POINT('Ctrl Pts',(-0.0743793001795075,-0.020114934867124,
-0.0611391236575861));
#51592=CARTESIAN_POINT('Ctrl Pts',(-0.0761392572294086,-0.0136071598667203,
-0.0616295434074734));
#51593=CARTESIAN_POINT('Ctrl Pts',(-0.076960594478556,-0.00684555435751792,
-0.0621199631573607));
#51594=CARTESIAN_POINT('Ctrl Pts',(-0.0769006083194561,-6.96495813230711E-5,
-0.062610382907248));
#51595=CARTESIAN_POINT('Ctrl Pts',(-0.0769139474189681,-7.03763467951925E-5,
-0.0676396170927522));
#51596=CARTESIAN_POINT('Ctrl Pts',(-0.0769713289242459,-0.00639183089268636,
-0.067181886303789));
#51597=CARTESIAN_POINT('Ctrl Pts',(-0.0762572933205676,-0.0127004960742668,
-0.0667241555148257));
#51598=CARTESIAN_POINT('Ctrl Pts',(-0.0747218360399382,-0.0188024656559839,
-0.0662664247258625));
#51599=CARTESIAN_POINT('Ctrl Pts',(-0.0685069541198702,-0.0435006587666868,
-0.0644137240089659));
#51600=CARTESIAN_POINT('Ctrl Pts',(-0.0488348182887464,-0.0648125823793867,
-0.0625610232920694));
#51601=CARTESIAN_POINT('Ctrl Pts',(-0.024712114252781,-0.0729807992742525,
-0.0607083225751728));
#51602=CARTESIAN_POINT('Ctrl Pts',(-0.000589410216815831,-0.0811490161691181,
-0.0588556218582763));
#51603=CARTESIAN_POINT('Ctrl Pts',(0.0279838620239908,-0.07617352634615,
-0.0570029211413797));
#51604=CARTESIAN_POINT('Ctrl Pts',(0.0479258495855115,-0.0603323589270951,
-0.0551502204244832));
#51605=CARTESIAN_POINT('Ctrl Pts',(0.0678678371470326,-0.0444911915080398,
-0.0532975197075866));
#51606=CARTESIAN_POINT('Ctrl Pts',(0.0791785400292676,-0.0177843464928974,
-0.0514448189906901));
#51607=CARTESIAN_POINT('Ctrl Pts',(0.0766793543706361,0.00756088938670773,
-0.0495921182737935));
#51608=CARTESIAN_POINT('Ctrl Pts',(0.0741801687120046,0.0329061252663129,
-0.047739417556897));
#51609=CARTESIAN_POINT('Ctrl Pts',(0.0578710945125066,0.0568897520103807,
-0.0458867168400004));
#51610=CARTESIAN_POINT('Ctrl Pts',(0.0352193012944682,0.0685309362054083,
-0.0440340161231038));
#51611=CARTESIAN_POINT('Ctrl Pts',(0.0125675080764302,0.0801721204004357,
-0.0421813154062073));
#51612=CARTESIAN_POINT('Ctrl Pts',(-0.0164270041601479,0.0794708620464232,
-0.0403286146893108));
#51613=CARTESIAN_POINT('Ctrl Pts',(-0.0384899414196672,0.0667486447887284,
-0.0384759139724143));
#51614=CARTESIAN_POINT('Ctrl Pts',(-0.0605528786791868,0.0540264275310334,
-0.0366232132555177));
#51615=CARTESIAN_POINT('Ctrl Pts',(-0.0756842409616474,0.0292832513696559,
-0.0347705125386211));
#51616=CARTESIAN_POINT('Ctrl Pts',(-0.0769553882282587,0.00384667954290156,
-0.0329178118217246));
#51617=CARTESIAN_POINT('Ctrl Pts',(-0.0770190118284969,0.00257352550336055,
-0.0328250802454004));
#51618=CARTESIAN_POINT('Ctrl Pts',(-0.0770479126307905,0.00129863435962909,
-0.0327323486690763));
#51619=CARTESIAN_POINT('Ctrl Pts',(-0.0770428135801558,2.35063928346054E-5,
-0.0326396170927521));
#51620=CARTESIAN_POINT('Origin',(0.,0.,-0.348563377523455));
#51621=CARTESIAN_POINT('',(-0.0570170345471334,1.21661208853844E-5,-0.0160633775234553));
#51622=CARTESIAN_POINT('',(-0.0568588689186872,3.50203243198108E-5,-0.00918662247654445));
#51623=CARTESIAN_POINT('',(-0.056925,-2.21215249084286E-15,-0.348563377523455));
#51624=CARTESIAN_POINT('',(0.0551371004056302,-0.0145210214852679,-9.0205620750794E-17));
#51625=CARTESIAN_POINT('Ctrl Pts',(-0.0570170345471334,1.21661208853871E-5,
-0.0160633775234553));
#51626=CARTESIAN_POINT('Ctrl Pts',(-0.0569658477122017,-0.0182269476124025,
-0.0142707194219589));
#51627=CARTESIAN_POINT('Ctrl Pts',(-0.0375869816080576,-0.0554112150194986,
-0.0106253606035659));
#51628=CARTESIAN_POINT('Ctrl Pts',(0.0240591212233117,-0.0619826963587815,
-0.00527090142908081));
#51629=CARTESIAN_POINT('Ctrl Pts',(0.0506098361506637,-0.0313215184444117,
-0.00170910035609219));
#51630=CARTESIAN_POINT('Ctrl Pts',(0.0551371004056302,-0.0145210214852679,
-9.23469200414528E-17));
#51631=CARTESIAN_POINT('',(0.00445734406721156,-0.056750222104116,0.));
#51632=CARTESIAN_POINT('Origin',(0.,0.,0.));
#51633=CARTESIAN_POINT('Ctrl Pts',(-0.0568588689186873,3.50203243198116E-5,
-0.00918662247654445));
#51634=CARTESIAN_POINT('Ctrl Pts',(-0.0567637403779411,-0.0123641010103422,
-0.00797711570125951));
#51635=CARTESIAN_POINT('Ctrl Pts',(-0.0466628848186406,-0.0438764064141307,
-0.00491490820907802));
#51636=CARTESIAN_POINT('Ctrl Pts',(-0.0144175559217569,-0.0582327171563943,
-0.0018527007168965));
#51637=CARTESIAN_POINT('Ctrl Pts',(0.00445734406721196,-0.0567502221041159,
5.55111512312578E-17));
#51638=CARTESIAN_POINT('Origin',(0.,0.,-0.348563377523455));
#51639=CARTESIAN_POINT('',(-0.0569069499978555,-5.15411428926268E-5,-0.0510633775234553));
#51640=CARTESIAN_POINT('',(-0.0570121828150844,1.7394883483156E-5,-0.0441866224765445));
#51641=CARTESIAN_POINT('',(-0.056925,-2.21215249084286E-15,-0.348563377523455));
#51642=CARTESIAN_POINT('Ctrl Pts',(-0.0569069499978555,-5.154114289264E-5,
-0.0510633775234553));
#51643=CARTESIAN_POINT('Ctrl Pts',(-0.0569513401454896,-0.00506575471955614,
-0.0505729577735681));
#51644=CARTESIAN_POINT('Ctrl Pts',(-0.0540474263512665,-0.0289720362496396,
-0.0482298373067843));
#51645=CARTESIAN_POINT('Ctrl Pts',(-0.0204550703512412,-0.0641028447178318,
-0.0440340161231039));
#51646=CARTESIAN_POINT('Ctrl Pts',(0.0427732686682708,-0.0519418462686033,
-0.0384759139724143));
#51647=CARTESIAN_POINT('Ctrl Pts',(0.0668367735916919,0.00778006570700472,
-0.0329178118217246));
#51648=CARTESIAN_POINT('Ctrl Pts',(0.0296964255967034,0.0603798012232959,
-0.027359709671035));
#51649=CARTESIAN_POINT('Ctrl Pts',(-0.0346304351480055,0.0576877321985291,
-0.0218016075203453));
#51650=CARTESIAN_POINT('Ctrl Pts',(-0.056734623549977,0.0200822897505687,
-0.0180361634711521));
#51651=CARTESIAN_POINT('Ctrl Pts',(-0.0570187489797074,0.000623060128065452,
-0.0161234201388554));
#51652=CARTESIAN_POINT('Ctrl Pts',(-0.0570170345471334,1.21661208853871E-5,
-0.0160633775234553));
#51653=CARTESIAN_POINT('Ctrl Pts',(-0.0570121828150844,1.73948834831544E-5,
-0.0441866224765445));
#51654=CARTESIAN_POINT('Ctrl Pts',(-0.0569405680998085,-0.017891414583955,
-0.0424266533359722));
#51655=CARTESIAN_POINT('Ctrl Pts',(-0.0381902384809938,-0.0547822163819881,
-0.0388139834785033));
#51656=CARTESIAN_POINT('Ctrl Pts',(0.0246325962628555,-0.0626129044013398,
-0.0333486129041379));
#51657=CARTESIAN_POINT('Ctrl Pts',(0.0659756148843137,-0.0132517004322241,
-0.0277905107534482));
#51658=CARTESIAN_POINT('Ctrl Pts',(0.0468879053916966,0.0482596214522584,
-0.0222324086027585));
#51659=CARTESIAN_POINT('Ctrl Pts',(-0.0150988217618111,0.0655506182074447,
-0.0166743064520689));
#51660=CARTESIAN_POINT('Ctrl Pts',(-0.0528320738248041,0.0321628305059058,
-0.0123257110766642));
#51661=CARTESIAN_POINT('Ctrl Pts',(-0.0569094565651003,0.00662864996470196,
-0.00982981641815606));
#51662=CARTESIAN_POINT('Ctrl Pts',(-0.0568588689186873,3.50203243198116E-5,
-0.00918662247654445));
#51663=CARTESIAN_POINT('Origin',(0.,0.,-0.348563377523455));
#51664=CARTESIAN_POINT('',(-0.0568373343912269,1.88788443762929E-5,-0.0860633775234553));
#51665=CARTESIAN_POINT('',(-0.0569168210181964,-5.20789540658581E-5,-0.0791866224765445));
#51666=CARTESIAN_POINT('',(-0.056925,-2.21215249084286E-15,-0.348563377523455));
#51667=CARTESIAN_POINT('Ctrl Pts',(-0.0568373343912269,1.88788443762919E-5,
-0.0860633775234553));
#51668=CARTESIAN_POINT('Ctrl Pts',(-0.0568055791606208,-0.0106562996884056,
-0.0850224954082807));
#51669=CARTESIAN_POINT('Ctrl Pts',(-0.0487872375507933,-0.0403768531512196,
-0.0821289125762096));
#51670=CARTESIAN_POINT('Ctrl Pts',(-0.000836488591294147,-0.0672820666389896,
-0.0773826290272417));
#51671=CARTESIAN_POINT('Ctrl Pts',(0.0560818346371597,-0.0371806680059875,
-0.0718245268765522));
#51672=CARTESIAN_POINT('Ctrl Pts',(0.0616474222580996,0.0269661419500831,
-0.0662664247258625));
#51673=CARTESIAN_POINT('Ctrl Pts',(0.0107639014093499,0.0664207519792408,
-0.0607083225751728));
#51674=CARTESIAN_POINT('Ctrl Pts',(-0.0446163690890475,0.0469405944497037,
-0.0556406401743705));
#51675=CARTESIAN_POINT('Ctrl Pts',(-0.0567836436806478,0.0138768696145832,
-0.0524256584904646));
#51676=CARTESIAN_POINT('Ctrl Pts',(-0.0569069499978555,-5.154114289264E-5,
-0.0510633775234553));
#51677=CARTESIAN_POINT('Ctrl Pts',(-0.0569168210181964,-5.2078954065865E-5,
-0.0791866224765445));
#51678=CARTESIAN_POINT('Ctrl Pts',(-0.0569592837050722,-0.00472999640645199,
-0.0787288916875813));
#51679=CARTESIAN_POINT('Ctrl Pts',(-0.0542921893886136,-0.0282943746581153,
-0.0764184601817215));
#51680=CARTESIAN_POINT('Ctrl Pts',(-0.0215805745713374,-0.0637326942294381,
-0.0722553279589653));
#51681=CARTESIAN_POINT('Ctrl Pts',(0.0418526469681333,-0.0526870098028222,
-0.0666972258082757));
#51682=CARTESIAN_POINT('Ctrl Pts',(0.0669626279198866,0.0066027069012525,
-0.061139123657586));
#51683=CARTESIAN_POINT('Ctrl Pts',(0.0307561651780042,0.0598468259421123,
-0.0555810215068964));
#51684=CARTESIAN_POINT('Ctrl Pts',(-0.0336122173660539,0.0582900187220077,
-0.0500229193562067));
#51685=CARTESIAN_POINT('Ctrl Pts',(-0.0565672790378523,0.0207533366878344,
-0.0462247863460895));
#51686=CARTESIAN_POINT('Ctrl Pts',(-0.0570159561456971,0.000960997867036193,
-0.0442793540528687));
#51687=CARTESIAN_POINT('Ctrl Pts',(-0.0570121828150844,1.73948834831544E-5,
-0.0441866224765445));
#51688=CARTESIAN_POINT('Origin',(0.,0.,-0.348563377523455));
#51689=CARTESIAN_POINT('',(-0.0569761128879509,4.19649640993781E-5,-0.121063377523455));
#51690=CARTESIAN_POINT('',(-0.0568344699801726,1.36387320454415E-5,-0.114186622476545));
#51691=CARTESIAN_POINT('',(-0.056925,-2.21215249084286E-15,-0.348563377523455));
#51692=CARTESIAN_POINT('Ctrl Pts',(-0.0569761128879509,4.19649640993761E-5,
-0.121063377523455));
#51693=CARTESIAN_POINT('Ctrl Pts',(-0.0568421140860372,-0.0161776865206131,
-0.119472033042993));
#51694=CARTESIAN_POINT('Ctrl Pts',(-0.041093804968909,-0.0515082139267437,
-0.116027987845635));
#51695=CARTESIAN_POINT('Ctrl Pts',(0.0188553037814868,-0.0645914338274078,
-0.110731241931379));
#51696=CARTESIAN_POINT('Ctrl Pts',(0.0644971261714122,-0.0191754133262199,
-0.10517313978069));
#51697=CARTESIAN_POINT('Ctrl Pts',(0.0510805017286943,0.0437990656879258,
-0.0996150376300002));
#51698=CARTESIAN_POINT('Ctrl Pts',(-0.00910929544596579,0.0666678078505591,
-0.0940569354793109));
#51699=CARTESIAN_POINT('Ctrl Pts',(-0.051248083903741,0.0356400444726433,
-0.0895397154437956));
#51700=CARTESIAN_POINT('Ctrl Pts',(-0.0568621013523766,0.00834480584732116,
-0.0868751961251772));
#51701=CARTESIAN_POINT('Ctrl Pts',(-0.0568373343912269,1.88788443762919E-5,
-0.0860633775234553));
#51702=CARTESIAN_POINT('Ctrl Pts',(-0.0568344699801726,1.36387320454363E-5,
-0.114186622476544));
#51703=CARTESIAN_POINT('Ctrl Pts',(-0.0568123121766602,-0.0103275848846827,
-0.113178429322294));
#51704=CARTESIAN_POINT('Ctrl Pts',(-0.0491635321171548,-0.0397028327409722,
-0.110317535451147));
#51705=CARTESIAN_POINT('Ctrl Pts',(-0.00202079792845361,-0.0672569095516575,
-0.105603940863103));
#51706=CARTESIAN_POINT('Ctrl Pts',(0.0554186211910062,-0.038162175403288,
-0.100045838712414));
#51707=CARTESIAN_POINT('Ctrl Pts',(0.0621125631276854,0.0258767294463682,
-0.0944877365617239));
#51708=CARTESIAN_POINT('Ctrl Pts',(0.0119315352940102,0.0662209506917629,
-0.0889296344110343));
#51709=CARTESIAN_POINT('Ctrl Pts',(-0.0441425466064682,0.047599427538858,
-0.0838292630493078));
#51710=CARTESIAN_POINT('Ctrl Pts',(-0.0567874127007329,0.0142042357374033,
-0.0805815924044779));
#51711=CARTESIAN_POINT('Ctrl Pts',(-0.0569168210181964,-5.2078954065865E-5,
-0.0791866224765445));
#51712=CARTESIAN_POINT('Origin',(0.,0.,-0.348563377523455));
#51713=CARTESIAN_POINT('',(-0.0569682917973646,-4.47457069638125E-5,-0.156063377523455));
#51714=CARTESIAN_POINT('',(-0.0569668622207115,4.51962923827109E-5,-0.149186622476545));
#51715=CARTESIAN_POINT('',(-0.056925,-2.21215249084286E-15,-0.348563377523455));
#51716=CARTESIAN_POINT('Ctrl Pts',(-0.0569682917973646,-4.4745706963804E-5,
-0.156063377523455));
#51717=CARTESIAN_POINT('Ctrl Pts',(-0.0569937221071028,-0.00299248950368808,
-0.155774271394602));
#51718=CARTESIAN_POINT('Ctrl Pts',(-0.0554451413155874,-0.0248036997598682,
-0.153632464548853));
#51719=CARTESIAN_POINT('Ctrl Pts',(-0.0272715619458597,-0.0615129069466198,
-0.149637956986207));
#51720=CARTESIAN_POINT('Ctrl Pts',(0.0369020781931099,-0.0562655523889355,
-0.144079854835517));
#51721=CARTESIAN_POINT('Ctrl Pts',(0.0672853847370649,0.000502797531543261,
-0.138521752684828));
#51722=CARTESIAN_POINT('Ctrl Pts',(0.0360571029361317,0.0568107482943974,
-0.132963650534138));
#51723=CARTESIAN_POINT('Ctrl Pts',(-0.0281877896808826,0.0610984803647731,
-0.127405548383449));
#51724=CARTESIAN_POINT('Ctrl Pts',(-0.0556177361256695,0.0242302520899051,
-0.123438790713221));
#51725=CARTESIAN_POINT('Ctrl Pts',(-0.0569981203307044,0.00270581752422716,
-0.12132473375989));
#51726=CARTESIAN_POINT('Ctrl Pts',(-0.0569761128879509,4.19649640993761E-5,
-0.121063377523455));
#51727=CARTESIAN_POINT('Ctrl Pts',(-0.0569668622207115,4.51962923827061E-5,
-0.149186622476545));
#51728=CARTESIAN_POINT('Ctrl Pts',(-0.0568288651124137,-0.0158479843568857,
-0.147627966957007));
#51729=CARTESIAN_POINT('Ctrl Pts',(-0.0416256884202204,-0.0508640579981459,
-0.144216610720572));
#51730=CARTESIAN_POINT('Ctrl Pts',(0.0177153124424513,-0.064913350971688,
-0.138952553767241));
#51731=CARTESIAN_POINT('Ctrl Pts',(0.0641495648705027,-0.0203078496210804,
-0.133394451616552));
#51732=CARTESIAN_POINT('Ctrl Pts',(0.0518436232068167,0.0428930549861271,
-0.127836349465862));
#51733=CARTESIAN_POINT('Ctrl Pts',(-0.00793426170214403,0.0668178339606645,
-0.122278247315172));
#51734=CARTESIAN_POINT('Ctrl Pts',(-0.0509215769942879,0.036317562629813,
-0.117728338318733));
#51735=CARTESIAN_POINT('Ctrl Pts',(-0.0568530303448794,0.00867590896718897,
-0.11503113003919));
#51736=CARTESIAN_POINT('Ctrl Pts',(-0.0568344699801726,1.36387320454363E-5,
-0.114186622476544));
#51737=CARTESIAN_POINT('Origin',(0.,0.,-0.348563377523455));
#51738=CARTESIAN_POINT('',(-0.0568348355527671,-1.44497151729769E-5,-0.191063377523455));
#51739=CARTESIAN_POINT('',(-0.0569774640760416,-4.14258005045076E-5,-0.184186622476544));
#51740=CARTESIAN_POINT('',(-0.056925,-2.21215249084286E-15,-0.348563377523455));
#51741=CARTESIAN_POINT('Ctrl Pts',(-0.056834835552767,-1.44497151729744E-5,
-0.191063377523455));
#51742=CARTESIAN_POINT('Ctrl Pts',(-0.0568543868502049,-0.00862591271069301,
-0.190223809029315));
#51743=CARTESIAN_POINT('Ctrl Pts',(-0.0509714490781074,-0.0362151985657714,
-0.187531539818278));
#51744=CARTESIAN_POINT('Ctrl Pts',(-0.00811195152116181,-0.0667965098284243,
-0.182986569890345));
#51745=CARTESIAN_POINT('Ctrl Pts',(0.0517293388381684,-0.0430308000507443,
-0.177428467739655));
#51746=CARTESIAN_POINT('Ctrl Pts',(0.0642033633612193,0.0201371382645114,
-0.171870365588966));
#51747=CARTESIAN_POINT('Ctrl Pts',(0.0178879160433239,0.0648660037698966,
-0.166312263438276));
#51748=CARTESIAN_POINT('Ctrl Pts',(-0.0415459569642868,0.0509615686075912,
-0.161043267416439));
#51749=CARTESIAN_POINT('Ctrl Pts',(-0.0568307551258429,0.0158977604785168,
-0.157626972111499));
#51750=CARTESIAN_POINT('Ctrl Pts',(-0.0569682917973646,-4.4745706963804E-5,
-0.156063377523455));
#51751=CARTESIAN_POINT('Ctrl Pts',(-0.0569774640760416,-4.14258005045011E-5,
-0.184186622476544));
#51752=CARTESIAN_POINT('Ctrl Pts',(-0.0569988598076398,-0.0026547751392027,
-0.183930205308616));
#51753=CARTESIAN_POINT('Ctrl Pts',(-0.0556479599452488,-0.0241282167988981,
-0.18182108742379));
#51754=CARTESIAN_POINT('Ctrl Pts',(-0.0283502073114013,-0.061023285478019,
-0.177859268822069));
#51755=CARTESIAN_POINT('Ctrl Pts',(0.0359058577506595,-0.0569064546902456,
-0.172301166671379));
#51756=CARTESIAN_POINT('Ctrl Pts',(0.0672838070486334,-0.000681773972618921,
-0.166743064520689));
#51757=CARTESIAN_POINT('Ctrl Pts',(0.0370516110423173,0.0561671930091792,
-0.161184962369999));
#51758=CARTESIAN_POINT('Ctrl Pts',(-0.0271078417631468,0.0615852280566224,
-0.15562686021931));
#51759=CARTESIAN_POINT('Ctrl Pts',(-0.0554139216188823,0.0249057972609597,
-0.151627413588158));
#51760=CARTESIAN_POINT('Ctrl Pts',(-0.0569928958031393,0.00304349410873103,
-0.149480667673903));
#51761=CARTESIAN_POINT('Ctrl Pts',(-0.0569668622207115,4.51962923827061E-5,
-0.149186622476545));
#51762=CARTESIAN_POINT('Origin',(0.,0.,-0.348563377523455));
#51763=CARTESIAN_POINT('',(-0.0569144593207152,5.12769584049947E-5,-0.226063377523455));
#51764=CARTESIAN_POINT('',(-0.0568377956013138,-1.97155662660445E-5,-0.219186622476544));
#51765=CARTESIAN_POINT('',(-0.056925,-2.21215249084286E-15,-0.348563377523455));
#51766=CARTESIAN_POINT('Ctrl Pts',(-0.0569144593207152,5.12769584049893E-5,
-0.226063377523455));
#51767=CARTESIAN_POINT('Ctrl Pts',(-0.056786042516509,-0.0141553962841083,
-0.224673346664028));
#51768=CARTESIAN_POINT('Ctrl Pts',(-0.0442160058077755,-0.0474988985344208,
-0.221430615087703));
#51769=CARTESIAN_POINT('Ctrl Pts',(0.011756104030695,-0.0662531338471764,
-0.216335182794483));
#51770=CARTESIAN_POINT('Ctrl Pts',(0.0620431155853323,-0.0260414998574271,
-0.210777080643793));
#51771=CARTESIAN_POINT('Ctrl Pts',(0.0555201480174088,0.0380144415731405,
-0.205218978493103));
#51772=CARTESIAN_POINT('Ctrl Pts',(-0.00184199994446337,0.0672621487551179,
-0.199660876342414));
#51773=CARTESIAN_POINT('Ctrl Pts',(-0.0491071931595563,0.0398046976257449,
-0.194942342685864));
#51774=CARTESIAN_POINT('Ctrl Pts',(-0.0568112424218084,0.0103772582952248,
-0.192076509746212));
#51775=CARTESIAN_POINT('Ctrl Pts',(-0.056834835552767,-1.44497151729744E-5,
-0.191063377523455));
#51776=CARTESIAN_POINT('Ctrl Pts',(-0.0568377956013138,-1.97155662660506E-5,
-0.219186622476544));
#51777=CARTESIAN_POINT('Ctrl Pts',(-0.0568634717455984,-0.00829475652583425,
-0.218379742943328));
#51778=CARTESIAN_POINT('Ctrl Pts',(-0.0512968444894828,-0.035537488922977,
-0.215720162693216));
#51779=CARTESIAN_POINT('Ctrl Pts',(-0.0092865044532633,-0.0666434551280208,
-0.211207881726207));
#51780=CARTESIAN_POINT('Ctrl Pts',(0.0509637654586514,-0.0439347205576348,
-0.205649779575517));
#51781=CARTESIAN_POINT('Ctrl Pts',(0.0645479274348034,0.0190037516412805,
-0.200091677424827));
#51782=CARTESIAN_POINT('Ctrl Pts',(0.0190270343003033,0.0645410651484606,
-0.194533575274137));
#51783=CARTESIAN_POINT('Ctrl Pts',(-0.0410125742824414,0.0516052793677545,
-0.189231890291377));
#51784=CARTESIAN_POINT('Ctrl Pts',(-0.0568442684142835,0.0162275572428938,
-0.185782906025512));
#51785=CARTESIAN_POINT('Ctrl Pts',(-0.0569774640760416,-4.14258005045011E-5,
-0.184186622476544));
#51786=CARTESIAN_POINT('Origin',(0.,0.,-0.348563377523455));
#51787=CARTESIAN_POINT('',(-0.056925,-2.21215249084286E-15,-0.2608));
#51788=CARTESIAN_POINT('',(-0.0569006472781276,4.53843407899977E-5,-0.254186622476544));
#51789=CARTESIAN_POINT('',(-0.056925,-2.21215249084286E-15,-0.348563377523455));
#51790=CARTESIAN_POINT('',(-0.0568613829974075,-0.00269049226390485,-0.2608));
#51791=CARTESIAN_POINT('Origin',(0.,0.,-0.2608));
#51792=CARTESIAN_POINT('Ctrl Pts',(-0.0568613829974075,-0.00269049226390492,
-0.2608));
#51793=CARTESIAN_POINT('Ctrl Pts',(-0.0559665358845781,-0.0216023639274464,
-0.258947299283104));
#51794=CARTESIAN_POINT('Ctrl Pts',(-0.0338414445280129,-0.0581356593406026,
-0.255241897849311));
#51795=CARTESIAN_POINT('Ctrl Pts',(0.030633014621353,-0.0599605699382118,
-0.249683795698621));
#51796=CARTESIAN_POINT('Ctrl Pts',(0.0669261363759389,-0.00676409500895024,
-0.244125693547931));
#51797=CARTESIAN_POINT('Ctrl Pts',(0.0420024582515309,0.0525667193079089,
-0.238567591397241));
#51798=CARTESIAN_POINT('Ctrl Pts',(-0.0214161385433601,0.0637944995354849,
-0.233009489246552));
#51799=CARTESIAN_POINT('Ctrl Pts',(-0.0542549075170614,0.0283960803383904,
-0.22884141795529));
#51800=CARTESIAN_POINT('Ctrl Pts',(-0.0569572026771635,0.00477994858439163,
-0.226526047380924));
#51801=CARTESIAN_POINT('Ctrl Pts',(-0.0569144593207152,5.12769584049893E-5,
-0.226063377523455));
#51802=CARTESIAN_POINT('Ctrl Pts',(-0.0569006472781276,4.53843407899985E-5,
-0.254186622476544));
#51803=CARTESIAN_POINT('Ctrl Pts',(-0.0567792970591674,-0.0138322573481857,
-0.252829280578041));
#51804=CARTESIAN_POINT('Ctrl Pts',(-0.04469426298412,-0.0468319938291516,
-0.249619237962641));
#51805=CARTESIAN_POINT('Ctrl Pts',(0.0105915237455798,-0.0664545630371273,
-0.244556494630344));
#51806=CARTESIAN_POINT('Ctrl Pts',(0.0615731857537621,-0.0271271707399214,
-0.238998392479655));
#51807=CARTESIAN_POINT('Ctrl Pts',(0.0561817391408256,0.0370298534016153,
-0.233440290328965));
#51808=CARTESIAN_POINT('Ctrl Pts',(-0.000658152491019542,0.067284844560902,
-0.227882188178275));
#51809=CARTESIAN_POINT('Ctrl Pts',(-0.0487294401428577,0.040478373884527,
-0.223130965560802));
#51810=CARTESIAN_POINT('Ctrl Pts',(-0.0568045159672386,0.0107058175214851,
-0.220232443660225));
#51811=CARTESIAN_POINT('Ctrl Pts',(-0.0568377956013138,-1.97155662660506E-5,
-0.219186622476544));
#51812=CARTESIAN_POINT('Ctrl Pts',(0.0565254421840274,-0.00673275656029344,
-0.272347005383792));
#51813=CARTESIAN_POINT('Ctrl Pts',(0.0587647304548727,0.0120673825140235,
-0.270494304666896));
#51814=CARTESIAN_POINT('Ctrl Pts',(0.0429739129313045,0.0517517526536903,
-0.266788903233103));
#51815=CARTESIAN_POINT('Ctrl Pts',(-0.0203148596464441,0.0641947008942669,
-0.261230801082414));
#51816=CARTESIAN_POINT('Ctrl Pts',(-0.0648913925766018,0.0177190613589564,
-0.255672698931723));
#51817=CARTESIAN_POINT('Ctrl Pts',(-0.0501036428777532,-0.0449120440985994,
-0.250114596781034));
#51818=CARTESIAN_POINT('Ctrl Pts',(0.0105915237455798,-0.0664545630371273,
-0.244556494630344));
#51819=CARTESIAN_POINT('Ctrl Pts',(0.0615731857537621,-0.0271271707399214,
-0.238998392479655));
#51820=CARTESIAN_POINT('Ctrl Pts',(0.0561817391408256,0.0370298534016153,
-0.233440290328965));
#51821=CARTESIAN_POINT('Ctrl Pts',(-0.000658152491019542,0.067284844560902,
-0.227882188178275));
#51822=CARTESIAN_POINT('Ctrl Pts',(-0.0568931784612784,0.03592594721713,
-0.222324086027586));
#51823=CARTESIAN_POINT('Ctrl Pts',(-0.0610336724629001,-0.0283279914129754,
-0.216765983876896));
#51824=CARTESIAN_POINT('Ctrl Pts',(-0.0092865044532633,-0.0666434551280208,
-0.211207881726207));
#51825=CARTESIAN_POINT('Ctrl Pts',(0.0509637654586514,-0.0439347205576348,
-0.205649779575517));
#51826=CARTESIAN_POINT('Ctrl Pts',(0.0645479274348034,0.0190037516412805,
-0.200091677424827));
#51827=CARTESIAN_POINT('Ctrl Pts',(0.0190270343003033,0.0645410651484606,
-0.194533575274137));
#51828=CARTESIAN_POINT('Ctrl Pts',(-0.0439164032436867,0.0509796372246231,
-0.188975473123448));
#51829=CARTESIAN_POINT('Ctrl Pts',(-0.0666466849838619,-0.00926257122266713,
-0.183417370972758));
#51830=CARTESIAN_POINT('Ctrl Pts',(-0.0283502073114013,-0.061023285478019,
-0.177859268822069));
#51831=CARTESIAN_POINT('Ctrl Pts',(0.0359058577506595,-0.0569064546902456,
-0.172301166671379));
#51832=CARTESIAN_POINT('Ctrl Pts',(0.0672838070486334,-0.000681773972618921,
-0.166743064520689));
#51833=CARTESIAN_POINT('Ctrl Pts',(0.0370516110423173,0.0561671930091792,
-0.161184962369999));
#51834=CARTESIAN_POINT('Ctrl Pts',(-0.0271078417631468,0.0615852280566224,
-0.15562686021931));
#51835=CARTESIAN_POINT('Ctrl Pts',(-0.0664453046257158,0.0106111703948657,
-0.15006875806862));
#51836=CARTESIAN_POINT('Ctrl Pts',(-0.0449404200929238,-0.0500792779013919,
-0.144510655917931));
#51837=CARTESIAN_POINT('Ctrl Pts',(0.0177153124424513,-0.064913350971688,
-0.138952553767241));
#51838=CARTESIAN_POINT('Ctrl Pts',(0.0641495648705027,-0.0203078496210804,
-0.133394451616552));
#51839=CARTESIAN_POINT('Ctrl Pts',(0.0518436232068167,0.0428930549861271,
-0.127836349465862));
#51840=CARTESIAN_POINT('Ctrl Pts',(-0.00793426170214403,0.0668178339606645,
-0.122278247315172));
#51841=CARTESIAN_POINT('Ctrl Pts',(-0.0604469360797266,0.029559149487349,
-0.116720145164483));
#51842=CARTESIAN_POINT('Ctrl Pts',(-0.0576098239656634,-0.0347661276820822,
-0.111162043013793));
#51843=CARTESIAN_POINT('Ctrl Pts',(-0.00202079792845361,-0.0672569095516575,
-0.105603940863103));
#51844=CARTESIAN_POINT('Ctrl Pts',(0.0554186211910062,-0.038162175403288,
-0.100045838712414));
#51845=CARTESIAN_POINT('Ctrl Pts',(0.0621125631276854,0.0258767294463682,
-0.0944877365617239));
#51846=CARTESIAN_POINT('Ctrl Pts',(0.0119315352940102,0.0662209506917629,
-0.0889296344110343));
#51847=CARTESIAN_POINT('Ctrl Pts',(-0.0491748926707758,0.045928246387533,
-0.0833715322603447));
#51848=CARTESIAN_POINT('Ctrl Pts',(-0.0652530997134914,-0.0164198082371239,
-0.0778134301096549));
#51849=CARTESIAN_POINT('Ctrl Pts',(-0.0215805745713374,-0.0637326942294381,
-0.0722553279589653));
#51850=CARTESIAN_POINT('Ctrl Pts',(0.0418526469681333,-0.0526870098028222,
-0.0666972258082757));
#51851=CARTESIAN_POINT('Ctrl Pts',(0.0669626279198866,0.0066027069012525,
-0.061139123657586));
#51852=CARTESIAN_POINT('Ctrl Pts',(0.0307561651780042,0.0598468259421123,
-0.0555810215068964));
#51853=CARTESIAN_POINT('Ctrl Pts',(-0.0336122173660539,0.0582900187220077,
-0.0500229193562067));
#51854=CARTESIAN_POINT('Ctrl Pts',(-0.0672041366873037,0.0033596851638767,
-0.0444648172055172));
#51855=CARTESIAN_POINT('Ctrl Pts',(-0.039256160803311,-0.054649352190282,
-0.0389067150548275));
#51856=CARTESIAN_POINT('Ctrl Pts',(0.0246325962628555,-0.0626129044013398,
-0.0333486129041379));
#51857=CARTESIAN_POINT('Ctrl Pts',(0.0659756148843137,-0.0132517004322241,
-0.0277905107534482));
#51858=CARTESIAN_POINT('Ctrl Pts',(0.0468879053916966,0.0482596214522584,
-0.0222324086027585));
#51859=CARTESIAN_POINT('Ctrl Pts',(-0.0150988217618111,0.0655506182074447,
-0.0166743064520689));
#51860=CARTESIAN_POINT('Ctrl Pts',(-0.0633271003986383,0.022876439855447,
-0.0111162043013792));
#51861=CARTESIAN_POINT('Ctrl Pts',(-0.0534357766767865,-0.0408609699628471,
-0.00555810215068963));
#51862=CARTESIAN_POINT('Ctrl Pts',(-0.0144175559217569,-0.0582327171563943,
-0.0018527007168965));
#51863=CARTESIAN_POINT('Ctrl Pts',(0.00445734406721196,-0.0567502221041159,
5.55111512312578E-17));
#51864=CARTESIAN_POINT('Ctrl Pts',(0.0631453153720265,-0.00752125096056229,
-0.268498003589195));
#51865=CARTESIAN_POINT('Ctrl Pts',(0.0656468537697459,0.0134806318203061,
-0.266645302872298));
#51866=CARTESIAN_POINT('Ctrl Pts',(0.0480067236976703,0.0578125639731092,
-0.262939901438505));
#51867=CARTESIAN_POINT('Ctrl Pts',(-0.0226939970666099,0.0717127452092156,
-0.257381799287816));
#51868=CARTESIAN_POINT('Ctrl Pts',(-0.0724910286564263,0.0197941966374174,
-0.251823697137126));
#51869=CARTESIAN_POINT('Ctrl Pts',(-0.0559714388523109,-0.0501718355316076,
-0.246265594986436));
#51870=CARTESIAN_POINT('Ctrl Pts',(0.0118319305669034,-0.0742372669501271,
-0.240707492835747));
#51871=CARTESIAN_POINT('Ctrl Pts',(0.0687842161450679,-0.0303041194431771,
-0.235149390685057));
#51872=CARTESIAN_POINT('Ctrl Pts',(0.0627613601791305,0.0413665365697152,
-0.229591288534368));
#51873=CARTESIAN_POINT('Ctrl Pts',(-0.000735230809393581,0.0751647853673317,
-0.224033186383678));
#51874=CARTESIAN_POINT('Ctrl Pts',(-0.0635561184069704,0.0401333484429689,
-0.218475084232988));
#51875=CARTESIAN_POINT('Ctrl Pts',(-0.068181518747532,-0.0316455720205553,
-0.212916982082299));
#51876=CARTESIAN_POINT('Ctrl Pts',(-0.0103740763406316,-0.0744482807907959,
-0.207358879931609));
#51877=CARTESIAN_POINT('Ctrl Pts',(0.0569322931071538,-0.0490800545418405,
-0.201800777780919));
#51878=CARTESIAN_POINT('Ctrl Pts',(0.0721073392263189,0.021229341059085,
-0.19624267563023));
#51879=CARTESIAN_POINT('Ctrl Pts',(0.0212553504238936,0.0720996732759336,
-0.19068457347954));
#51880=CARTESIAN_POINT('Ctrl Pts',(-0.0490595920293621,0.0569500236658029,
-0.18512647132885));
#51881=CARTESIAN_POINT('Ctrl Pts',(-0.0744518889052628,-0.0103473402137565,
-0.179568369178161));
#51882=CARTESIAN_POINT('Ctrl Pts',(-0.0316703896930619,-0.0681699153100223,
-0.174010267027471));
#51883=CARTESIAN_POINT('Ctrl Pts',(0.040110906235585,-0.0635709494570729,
-0.168452164876781));
#51884=CARTESIAN_POINT('Ctrl Pts',(0.0751636263487222,-0.000761618677361565,
-0.162894062726092));
#51885=CARTESIAN_POINT('Ctrl Pts',(0.0413908423164874,0.0627451105040324,
-0.157335960575402));
#51886=CARTESIAN_POINT('Ctrl Pts',(-0.0302825267888408,0.068797668760077,
-0.151777858424713));
#51887=CARTESIAN_POINT('Ctrl Pts',(-0.0742269242568931,0.0118538780973828,
-0.146219756274023));
#51888=CARTESIAN_POINT('Ctrl Pts',(-0.0502035347283126,-0.0559442204165597,
-0.140661654123333));
#51889=CARTESIAN_POINT('Ctrl Pts',(0.0197900086734511,-0.0725155586685627,
-0.135103551972644));
#51890=CARTESIAN_POINT('Ctrl Pts',(0.0716623231630515,-0.0226861660750207,
-0.129545449821954));
#51891=CARTESIAN_POINT('Ctrl Pts',(0.057915193777078,0.0479163962229738,
-0.123987347671264));
#51892=CARTESIAN_POINT('Ctrl Pts',(-0.00886346816704126,0.0746430816796707,
-0.118429245520575));
#51893=CARTESIAN_POINT('Ctrl Pts',(-0.067526067812091,0.033020914908207,
-0.112871143369885));
#51894=CARTESIAN_POINT('Ctrl Pts',(-0.0643566925313977,-0.0388376987764555,
-0.107313041219195));
#51895=CARTESIAN_POINT('Ctrl Pts',(-0.0022574599607718,-0.0751335788008634,
-0.101754939068506));
#51896=CARTESIAN_POINT('Ctrl Pts',(0.0619088710743035,-0.0426314683798115,
-0.0961968369178161));
#51897=CARTESIAN_POINT('Ctrl Pts',(0.0693867617080029,0.0289072350176012,
-0.0906387347671264));
#51898=CARTESIAN_POINT('Ctrl Pts',(0.0133288751030001,0.0739762955246439,
-0.0850806326164367));
#51899=CARTESIAN_POINT('Ctrl Pts',(-0.0549339197731941,0.0513070484823988,
-0.0795225304657472));
#51900=CARTESIAN_POINT('Ctrl Pts',(-0.0728950964593256,-0.0183427838760783,
-0.0739644283150574));
#51901=CARTESIAN_POINT('Ctrl Pts',(-0.0241079438667659,-0.0711966314836541,
-0.0684063261643679));
#51902=CARTESIAN_POINT('Ctrl Pts',(0.0467541427336881,-0.0588573520429421,
-0.0628482240136781));
#51903=CARTESIAN_POINT('Ctrl Pts',(0.0748048329170919,0.00737597077491671,
-0.0572901218629886));
#51904=CARTESIAN_POINT('Ctrl Pts',(0.0343581168896724,0.0668556768795576,
-0.0517320197122989));
#51905=CARTESIAN_POINT('Ctrl Pts',(-0.0375486503762781,0.0651165470454754,
-0.0461739175616092));
#51906=CARTESIAN_POINT('Ctrl Pts',(-0.0750746255395717,0.00375314851201067,
-0.0406158154109196));
#51907=CARTESIAN_POINT('Ctrl Pts',(-0.0438535738676721,-0.0610495105495594,
-0.03505771326023));
#51908=CARTESIAN_POINT('Ctrl Pts',(0.0275173974647707,-0.0699456995295894,
-0.0294996111095403));
#51909=CARTESIAN_POINT('Ctrl Pts',(0.0737022276653781,-0.0148036489530528,
-0.0239415089588508));
#51910=CARTESIAN_POINT('Ctrl Pts',(0.05237909618563,0.0539114582494777,
-0.018383406808161));
#51911=CARTESIAN_POINT('Ctrl Pts',(-0.016867092499543,0.0732274582844401,
-0.0128253046574715));
#51912=CARTESIAN_POINT('Ctrl Pts',(-0.0707435372774131,0.0255555720299983,
-0.00726720250678171));
#51913=CARTESIAN_POINT('Ctrl Pts',(-0.0596938093720625,-0.0456463273000271,
-0.00170910035609216));
#51914=CARTESIAN_POINT('Ctrl Pts',(-0.0161060414637576,-0.0650525347124059,
0.001996301077701));
#51915=CARTESIAN_POINT('Ctrl Pts',(0.00497935771876632,-0.0633964199789941,
0.00384900179459755));
#51916=CARTESIAN_POINT('Ctrl Pts',(0.0697651885600256,-0.00830974536083114,
-0.264649001794597));
#51917=CARTESIAN_POINT('Ctrl Pts',(0.072528977084619,0.0148938811265888,
-0.262796301077701));
#51918=CARTESIAN_POINT('Ctrl Pts',(0.0530395344640362,0.0638733752925282,
-0.259090899643908));
#51919=CARTESIAN_POINT('Ctrl Pts',(-0.0250731344867759,0.0792307895241642,
-0.253532797493218));
#51920=CARTESIAN_POINT('Ctrl Pts',(-0.0800906647362507,0.0218693319158784,
-0.247974695342528));
#51921=CARTESIAN_POINT('Ctrl Pts',(-0.0618392348268687,-0.0554316269646156,
-0.242416593191839));
#51922=CARTESIAN_POINT('Ctrl Pts',(0.0130723373882271,-0.082019970863127,
-0.236858491041149));
#51923=CARTESIAN_POINT('Ctrl Pts',(0.0759952465363734,-0.0334810681464326,
-0.23130038889046));
#51924=CARTESIAN_POINT('Ctrl Pts',(0.0693409812174357,0.045703219737815,
-0.22574228673977));
#51925=CARTESIAN_POINT('Ctrl Pts',(-0.000812309127767784,0.0830447261737616,
-0.22018418458908));
#51926=CARTESIAN_POINT('Ctrl Pts',(-0.0702190583526623,0.0443407496688078,
-0.214626082438391));
#51927=CARTESIAN_POINT('Ctrl Pts',(-0.0753293650321641,-0.0349631526281352,
-0.209067980287701));
#51928=CARTESIAN_POINT('Ctrl Pts',(-0.0114616482279998,-0.0822531064535709,
-0.203509878137011));
#51929=CARTESIAN_POINT('Ctrl Pts',(0.0629008207556561,-0.0542253885260463,
-0.197951775986322));
#51930=CARTESIAN_POINT('Ctrl Pts',(0.0796667510178346,0.0234549304768895,
-0.192393673835632));
#51931=CARTESIAN_POINT('Ctrl Pts',(0.0234836665474837,0.0796582814034065,
-0.186835571684942));
#51932=CARTESIAN_POINT('Ctrl Pts',(-0.0542027808150372,0.0629204101069829,
-0.181277469534253));
#51933=CARTESIAN_POINT('Ctrl Pts',(-0.0822570928266639,-0.011432109204846,
-0.175719367383563));
#51934=CARTESIAN_POINT('Ctrl Pts',(-0.0349905720747223,-0.0753165451420255,
-0.170161265232874));
#51935=CARTESIAN_POINT('Ctrl Pts',(0.0443159547205104,-0.0702354442239004,
-0.164603163082184));
#51936=CARTESIAN_POINT('Ctrl Pts',(0.0830434456488111,-0.000841463382104197,
-0.159045060931494));
#51937=CARTESIAN_POINT('Ctrl Pts',(0.0457300735906574,0.0693230279988856,
-0.153486958780804));
#51938=CARTESIAN_POINT('Ctrl Pts',(-0.0334572118145347,0.0760101094635317,
-0.147928856630115));
#51939=CARTESIAN_POINT('Ctrl Pts',(-0.0820085438880705,0.0130965857998999,
-0.142370754479425));
#51940=CARTESIAN_POINT('Ctrl Pts',(-0.0554666493637013,-0.0618091629317276,
-0.136812652328736));
#51941=CARTESIAN_POINT('Ctrl Pts',(0.0218647049044507,-0.0801177663654375,
-0.131254550178046));
#51942=CARTESIAN_POINT('Ctrl Pts',(0.0791750814556004,-0.0250644825289609,
-0.125696448027356));
#51943=CARTESIAN_POINT('Ctrl Pts',(0.0639867643473392,0.0529397374598205,
-0.120138345876667));
#51944=CARTESIAN_POINT('Ctrl Pts',(-0.0097926746319385,0.0824683293986771,
-0.114580243725977));
#51945=CARTESIAN_POINT('Ctrl Pts',(-0.0746051995444553,0.036482680329065,
-0.109022141575287));
#51946=CARTESIAN_POINT('Ctrl Pts',(-0.0711035610971321,-0.0429092698708288,
-0.103464039424598));
#51947=CARTESIAN_POINT('Ctrl Pts',(-0.00249412199308987,-0.0830102480500694,
-0.0979059372739083));
#51948=CARTESIAN_POINT('Ctrl Pts',(0.0683991209576008,-0.047100761356335,
-0.0923478351232185));
#51949=CARTESIAN_POINT('Ctrl Pts',(0.0766609602883205,0.0319377405888342,
-0.0867897329725289));
#51950=CARTESIAN_POINT('Ctrl Pts',(0.01472621491199,0.0817316403575249,
-0.0812316308218393));
#51951=CARTESIAN_POINT('Ctrl Pts',(-0.0606929468756124,0.0566858505772645,
-0.0756735286711496));
#51952=CARTESIAN_POINT('Ctrl Pts',(-0.0805370932051599,-0.0202657595150326,
-0.07011542652046));
#51953=CARTESIAN_POINT('Ctrl Pts',(-0.0266353131621943,-0.0786605687378701,
-0.0645573243697703));
#51954=CARTESIAN_POINT('Ctrl Pts',(0.0516556384992429,-0.065027694283062,
-0.0589992222190807));
#51955=CARTESIAN_POINT('Ctrl Pts',(0.0826470379142973,0.00814923464858084,
-0.053441120068391));
#51956=CARTESIAN_POINT('Ctrl Pts',(0.0379600686013405,0.073864527817003,
-0.0478830179177014));
#51957=CARTESIAN_POINT('Ctrl Pts',(-0.0414850833865023,0.071943075368943,
-0.0423249157670118));
#51958=CARTESIAN_POINT('Ctrl Pts',(-0.0829451143918398,0.00414661186014473,
-0.0367668136163221));
#51959=CARTESIAN_POINT('Ctrl Pts',(-0.0484509869320331,-0.0674496689088369,
-0.0312087114656326));
#51960=CARTESIAN_POINT('Ctrl Pts',(0.0304021986666858,-0.0772784946578389,
-0.0256506093149427));
#51961=CARTESIAN_POINT('Ctrl Pts',(0.0814288404464425,-0.0163555974738817,
-0.0200925071642533));
#51962=CARTESIAN_POINT('Ctrl Pts',(0.0578702869795633,0.0595632950466971,
-0.0145344050135635));
#51963=CARTESIAN_POINT('Ctrl Pts',(-0.0186353632372748,0.0809042983614356,
-0.00897630286287398));
#51964=CARTESIAN_POINT('Ctrl Pts',(-0.0781599741561879,0.0282347042045496,
-0.00341820071218422));
#51965=CARTESIAN_POINT('Ctrl Pts',(-0.0659518420673384,-0.050431684637207,
0.00213990143850535));
#51966=CARTESIAN_POINT('Ctrl Pts',(-0.0177945270057585,-0.0718723522684174,
0.0058453028722985));
#51967=CARTESIAN_POINT('Ctrl Pts',(0.00550137137032068,-0.0700426178538723,
0.00769800358919505));
#51968=CARTESIAN_POINT('Ctrl Pts',(0.0763850617480246,-0.00909823976109999,
-0.2608));
#51969=CARTESIAN_POINT('Ctrl Pts',(0.0794111003994922,0.0163071304328715,
-0.258947299283103));
#51970=CARTESIAN_POINT('Ctrl Pts',(0.058072345230402,0.0699341866119471,
-0.25524189784931));
#51971=CARTESIAN_POINT('Ctrl Pts',(-0.0274522719069417,0.086748833839113,
-0.249683795698621));
#51972=CARTESIAN_POINT('Ctrl Pts',(-0.0876903008160753,0.0239444671943393,
-0.244125693547931));
#51973=CARTESIAN_POINT('Ctrl Pts',(-0.0677070308014264,-0.0606914183976236,
-0.238567591397241));
#51974=CARTESIAN_POINT('Ctrl Pts',(0.0143127442095507,-0.089802674776127,
-0.233009489246552));
#51975=CARTESIAN_POINT('Ctrl Pts',(0.0832062769276791,-0.0366580168496882,
-0.227451387095862));
#51976=CARTESIAN_POINT('Ctrl Pts',(0.0759206022557407,0.0500399029059149,
-0.221893284945172));
#51977=CARTESIAN_POINT('Ctrl Pts',(-0.000889387446141895,0.0909246669801913,
-0.216335182794483));
#51978=CARTESIAN_POINT('Ctrl Pts',(-0.0768819982983542,0.0485481508946467,
-0.210777080643793));
#51979=CARTESIAN_POINT('Ctrl Pts',(-0.0824772113167961,-0.038280733235715,
-0.205218978493104));
#51980=CARTESIAN_POINT('Ctrl Pts',(-0.0125492201153681,-0.0900579321163461,
-0.199660876342414));
#51981=CARTESIAN_POINT('Ctrl Pts',(0.0688693484041585,-0.0593707225102519,
-0.194102774191724));
#51982=CARTESIAN_POINT('Ctrl Pts',(0.0872261628093503,0.0256805198946939,
-0.188544672041035));
#51983=CARTESIAN_POINT('Ctrl Pts',(0.025711982671074,0.0872168895308795,
-0.182986569890345));
#51984=CARTESIAN_POINT('Ctrl Pts',(-0.0593459696007125,0.0688907965481627,
-0.177428467739655));
#51985=CARTESIAN_POINT('Ctrl Pts',(-0.0900622967480648,-0.0125168781959353,
-0.171870365588966));
#51986=CARTESIAN_POINT('Ctrl Pts',(-0.0383107544563828,-0.0824631749740288,
-0.166312263438276));
#51987=CARTESIAN_POINT('Ctrl Pts',(0.0485210032054359,-0.0768999389907277,
-0.160754161287586));
#51988=CARTESIAN_POINT('Ctrl Pts',(0.0909232649488999,-0.000921308086846913,
-0.155196059136897));
#51989=CARTESIAN_POINT('Ctrl Pts',(0.0500693048648274,0.0759009454937388,
-0.149637956986207));
#51990=CARTESIAN_POINT('Ctrl Pts',(-0.0366318968402287,0.0832225501669864,
-0.144079854835518));
#51991=CARTESIAN_POINT('Ctrl Pts',(-0.0897901635192477,0.0143392935024171,
-0.138521752684828));
#51992=CARTESIAN_POINT('Ctrl Pts',(-0.0607297639990901,-0.0676741054468955,
-0.132963650534138));
#51993=CARTESIAN_POINT('Ctrl Pts',(0.0239394011354505,-0.0877199740623122,
-0.127405548383449));
#51994=CARTESIAN_POINT('Ctrl Pts',(0.0866878397481493,-0.0274427989829012,
-0.121847446232759));
#51995=CARTESIAN_POINT('Ctrl Pts',(0.0700583349176005,0.0579630786966672,
-0.116289344082069));
#51996=CARTESIAN_POINT('Ctrl Pts',(-0.0107218810968358,0.0902935771176834,
-0.11073124193138));
#51997=CARTESIAN_POINT('Ctrl Pts',(-0.0816843312768195,0.039944445749923,
-0.10517313978069));
#51998=CARTESIAN_POINT('Ctrl Pts',(-0.0778504296628665,-0.0469808409652021,
-0.0996150376300002));
#51999=CARTESIAN_POINT('Ctrl Pts',(-0.002730784025408,-0.0908869172992753,
-0.0940569354793109));
#52000=CARTESIAN_POINT('Ctrl Pts',(0.0748893708408981,-0.0515700543328586,
-0.0884988333286209));
#52001=CARTESIAN_POINT('Ctrl Pts',(0.083935158868638,0.0349682461600672,
-0.0829407311779315));
#52002=CARTESIAN_POINT('Ctrl Pts',(0.01612355472098,0.0894869851904058,
-0.0773826290272417));
#52003=CARTESIAN_POINT('Ctrl Pts',(-0.0664519739780307,0.0620646526721303,
-0.0718245268765522));
#52004=CARTESIAN_POINT('Ctrl Pts',(-0.088179089950994,-0.022188735153987,
-0.0662664247258625));
#52005=CARTESIAN_POINT('Ctrl Pts',(-0.0291626824576228,-0.0861245059920862,
-0.0607083225751728));
#52006=CARTESIAN_POINT('Ctrl Pts',(0.0565571342647977,-0.0711980365231819,
-0.0551502204244832));
#52007=CARTESIAN_POINT('Ctrl Pts',(0.0904892429115026,0.00892249852224505,
-0.0495921182737936));
#52008=CARTESIAN_POINT('Ctrl Pts',(0.0415620203130087,0.0808733787544482,
-0.0440340161231039));
#52009=CARTESIAN_POINT('Ctrl Pts',(-0.0454215163967265,0.0787696036924106,
-0.0384759139724143));
#52010=CARTESIAN_POINT('Ctrl Pts',(-0.0908156032441078,0.00454007520827874,
-0.0329178118217246));
#52011=CARTESIAN_POINT('Ctrl Pts',(-0.0530483999963943,-0.0738498272681144,
-0.0273597096710351));
#52012=CARTESIAN_POINT('Ctrl Pts',(0.0332869998686011,-0.0846112897860884,
-0.0218016075203453));
#52013=CARTESIAN_POINT('Ctrl Pts',(0.0891554532275068,-0.0179075459947105,
-0.0162435053696558));
#52014=CARTESIAN_POINT('Ctrl Pts',(0.0633614777734967,0.0652151318439164,
-0.010685403218966));
#52015=CARTESIAN_POINT('Ctrl Pts',(-0.0204036339750069,0.0885811384384311,
-0.00512730106827648));
#52016=CARTESIAN_POINT('Ctrl Pts',(-0.0855764110349624,0.0309138363791009,
0.00043080108241328));
#52017=CARTESIAN_POINT('Ctrl Pts',(-0.0722098747626145,-0.0552170419743869,
0.00598890323310284));
#52018=CARTESIAN_POINT('Ctrl Pts',(-0.0194830125477592,-0.078692169824429,
0.00969430466689599));
#52019=CARTESIAN_POINT('Ctrl Pts',(0.00602338502187503,-0.0766888157287505,
0.0115470053837926));
#52020=CARTESIAN_POINT('',(-0.0702475453412058,0.0316531309938693,3.81639164714898E-17));
#52021=CARTESIAN_POINT('Ctrl Pts',(-0.0702475453412056,0.0316531309938698,
1.04083408558608E-17));
#52022=CARTESIAN_POINT('Ctrl Pts',(-0.0708401438323926,0.029761073498479,
5.79235680573455E-18));
#52023=CARTESIAN_POINT('Ctrl Pts',(-0.0713533641733164,0.0278477587888483,
-2.19516502096945E-17));
#52024=CARTESIAN_POINT('Ctrl Pts',(-0.0717834091387127,0.0259160599661846,
-5.03069808033274E-17));
#52025=CARTESIAN_POINT('Ctrl Pts',(-0.0726956731599413,0.0218183039695723,
-1.10399493300004E-16));
#52026=CARTESIAN_POINT('Ctrl Pts',(-0.0732342513009639,0.0176375932737427,
-1.2801402186765E-16));
#52027=CARTESIAN_POINT('Ctrl Pts',(-0.0734091543575676,0.0134222320461422,
-1.14491749414469E-16));
#52028=CARTESIAN_POINT('Ctrl Pts',(-0.0735212566871715,0.0107204392764101,
-1.05824786852604E-16));
#52029=CARTESIAN_POINT('Ctrl Pts',(-0.0734832703910439,0.00800545788437908,
-8.75273381590973E-17));
#52030=CARTESIAN_POINT('Ctrl Pts',(-0.0732984068112228,0.00530313201976544,
-9.54097911787244E-17));
#52031=CARTESIAN_POINT('Ctrl Pts',(-0.0729691788812362,0.000490495850885873,
-1.09447838550622E-16));
#52032=CARTESIAN_POINT('Ctrl Pts',(-0.0721756952260308,-0.00429375429852149,
-1.18695651748223E-16));
#52033=CARTESIAN_POINT('Ctrl Pts',(-0.0709276079677427,-0.00897089557555983,
-9.54097911787244E-17));
#52034=CARTESIAN_POINT('Ctrl Pts',(-0.0703102811078677,-0.0112842954749435,
-8.38921772543806E-17));
#52035=CARTESIAN_POINT('Ctrl Pts',(-0.0695840020575365,-0.0135618869643576,
-1.04445390710516E-16));
#52036=CARTESIAN_POINT('Ctrl Pts',(-0.0687513992021191,-0.0157936705084804,
-1.04083408558608E-16));
#52037=CARTESIAN_POINT('Ctrl Pts',(-0.0667739557564809,-0.0210941876910649,
-1.03223695876781E-16));
#52038=CARTESIAN_POINT('Ctrl Pts',(-0.0641981025339425,-0.0261408913163681,
-4.81033231372627E-17));
#52039=CARTESIAN_POINT('Ctrl Pts',(-0.0610330648987858,-0.0307922157670597,
-4.85722573273506E-17));
#52040=CARTESIAN_POINT('Ctrl Pts',(-0.0595995290513461,-0.0328989333188744,
-4.87846510013196E-17));
#52041=CARTESIAN_POINT('Ctrl Pts',(-0.0580434790487478,-0.034924535640895,
-9.75325019484706E-17));
#52042=CARTESIAN_POINT('Ctrl Pts',(-0.0563782123517984,-0.036839591092707,
-8.32667268468867E-17));
#52043=CARTESIAN_POINT('Ctrl Pts',(-0.055297679654866,-0.0380822028833062,
-7.40101696404141E-17));
#52044=CARTESIAN_POINT('Ctrl Pts',(-0.0541700936089916,-0.0392799543399077,
-3.01247228678535E-17));
#52045=CARTESIAN_POINT('Ctrl Pts',(-0.0529957554081263,-0.0404291985015901,
-3.81639164714898E-17));
#52046=CARTESIAN_POINT('Ctrl Pts',(-0.0507006751620624,-0.0426752359475643,
-5.38753992627271E-17));
#52047=CARTESIAN_POINT('Ctrl Pts',(-0.0482270615803998,-0.0447363204158576,
-9.98006814252804E-17));
#52048=CARTESIAN_POINT('Ctrl Pts',(-0.0456008459049946,-0.0466020203916923,
-8.41340885848751E-17));
#52049=CARTESIAN_POINT('Ctrl Pts',(-0.0437719639308629,-0.0479012834670357,
-7.32239605591342E-17));
#52050=CARTESIAN_POINT('Ctrl Pts',(-0.0418673313980074,-0.0491066227264505,
-6.15450822730729E-17));
#52051=CARTESIAN_POINT('Ctrl Pts',(-0.0399010703140815,-0.0502099840408421,
-5.20417042793042E-17));
#52052=CARTESIAN_POINT('Ctrl Pts',(-0.0351580807136298,-0.0528714979580334,
-2.91177785798691E-17));
#52053=CARTESIAN_POINT('Ctrl Pts',(-0.0300947711453647,-0.0549234116843586,
-7.62798734692924E-18));
#52054=CARTESIAN_POINT('Ctrl Pts',(-0.0248427491906684,-0.0563131705928901,
3.51281503885303E-17));
#52055=CARTESIAN_POINT('Ctrl Pts',(-0.0227105540742067,-0.0568773794220593,
5.24861182082942E-17));
#52056=CARTESIAN_POINT('Ctrl Pts',(-0.0205472623921807,-0.0573318683473704,
-3.01179988497144E-17));
#52057=CARTESIAN_POINT('Ctrl Pts',(-0.0183622887047919,-0.0576706893152479,
-2.55871712706579E-17));
#52058=CARTESIAN_POINT('Ctrl Pts',(-0.0161895643360923,-0.0580076107975444,
-2.10817442496316E-17));
#52059=CARTESIAN_POINT('Ctrl Pts',(-0.0140040937456036,-0.058228676608621,
-6.10708131189109E-17));
#52060=CARTESIAN_POINT('Ctrl Pts',(-0.0118192148552885,-0.058329734875705,
-5.48606299277665E-17));
#52061=CARTESIAN_POINT('Ctrl Pts',(-0.0068511720320565,-0.0585595241792404,
-4.07397300598246E-17));
#52062=CARTESIAN_POINT('Ctrl Pts',(-0.00187688283265028,-0.058172909763502,
7.5769660385224E-17));
#52063=CARTESIAN_POINT('Ctrl Pts',(0.00298509850992475,-0.0570979057708017,
3.98444298388423E-17));
#52064=CARTESIAN_POINT('Ctrl Pts',(0.00347707029304418,-0.0569891287941157,
3.62092452329056E-17));
#52065=CARTESIAN_POINT('Ctrl Pts',(0.00396786625890273,-0.0568732671910623,
5.43496127043497E-17));
#52066=CARTESIAN_POINT('Ctrl Pts',(0.00445734406721196,-0.0567502221041159,
5.46437894932694E-17));
#52067=CARTESIAN_POINT('Ctrl Pts',(-0.0770428135801558,2.35063928346054E-5,
-0.0326396170927521));
#52068=CARTESIAN_POINT('Ctrl Pts',(-0.0769460377879284,-0.0241773749120882,
-0.0308796479521797));
#52069=CARTESIAN_POINT('Ctrl Pts',(-0.0646022015971733,-0.0484635620670927,
-0.0291196788116074));
#52070=CARTESIAN_POINT('Ctrl Pts',(-0.044953700560181,-0.0625784206083777,
-0.027359709671035));
#52071=CARTESIAN_POINT('Ctrl Pts',(-0.0242699333747295,-0.0774369814407723,
-0.0255070089541385));
#52072=CARTESIAN_POINT('Ctrl Pts',(0.00450853324693592,-0.0810241356134303,
-0.0236543082372419));
#52073=CARTESIAN_POINT('Ctrl Pts',(0.0282091754509194,-0.071700422067863,
-0.0218016075203453));
#52074=CARTESIAN_POINT('Ctrl Pts',(0.0519098176549031,-0.0623767085222956,
-0.0199489068034488));
#52075=CARTESIAN_POINT('Ctrl Pts',(0.070532635441205,-0.040142127258503,
-0.0180962060865523));
#52076=CARTESIAN_POINT('Ctrl Pts',(0.0755450484253542,-0.0151710569868353,
-0.0162435053696557));
#52077=CARTESIAN_POINT('Ctrl Pts',(0.0805574614095034,0.00980001328483202,
-0.0143908046527592));
#52078=CARTESIAN_POINT('Ctrl Pts',(0.0719594695915001,0.0375075725643739,
-0.0125381039358626));
#52079=CARTESIAN_POINT('Ctrl Pts',(0.0536996217244147,0.0552556866365642,
-0.0106854032189661));
#52080=CARTESIAN_POINT('Ctrl Pts',(0.0354397738573291,0.0730038007087545,
-0.0088327025020695));
#52081=CARTESIAN_POINT('Ctrl Pts',(0.00751806994116074,0.0807924695735928,
-0.00698000178517297));
#52082=CARTESIAN_POINT('Ctrl Pts',(-0.0173049115269158,0.0750755869961235,
-0.00512730106827642));
#52083=CARTESIAN_POINT('Ctrl Pts',(-0.0402038968187358,0.0698018123601118,
-0.00341820071218428));
#52084=CARTESIAN_POINT('Ctrl Pts',(-0.0604658994839416,0.0530349449696514,
-0.00170910035609212));
#52085=CARTESIAN_POINT('Ctrl Pts',(-0.0702475453412058,0.0316531309938693,
3.81639164714898E-17));
#52086=CARTESIAN_POINT('',(-0.0213030042343867,0.0527886127454558,-0.2608));
#52087=CARTESIAN_POINT('Ctrl Pts',(-0.0213170383639363,0.0528823612671138,
-0.2608));
#52088=CARTESIAN_POINT('Ctrl Pts',(-0.0200481268693847,0.0536735018248238,
-0.2608));
#52089=CARTESIAN_POINT('Ctrl Pts',(-0.0187486983558779,0.0544095042513574,
-0.2608));
#52090=CARTESIAN_POINT('Ctrl Pts',(-0.0174215591439766,0.0550876795506691,
-0.2608));
#52091=CARTESIAN_POINT('Ctrl Pts',(-0.0145506047994946,0.0565547527140716,
-0.2608));
#52092=CARTESIAN_POINT('Ctrl Pts',(-0.0115504229589048,0.0577517065377783,
-0.2608));
#52093=CARTESIAN_POINT('Ctrl Pts',(-0.00845775334810257,0.0586900169041967,
-0.2608));
#52094=CARTESIAN_POINT('Ctrl Pts',(-0.00612165927441171,0.0593987836210216,
-0.2608));
#52095=CARTESIAN_POINT('Ctrl Pts',(-0.00373424326947691,0.0599588209332557,
-0.2608));
#52096=CARTESIAN_POINT('Ctrl Pts',(-0.0013224230181328,0.0603724403993434,
-0.2608));
#52097=CARTESIAN_POINT('Ctrl Pts',(0.00185366586643284,0.0609171294937934,
-0.2608));
#52098=CARTESIAN_POINT('Ctrl Pts',(0.00507722273770718,0.0612098644046175,
-0.2608));
#52099=CARTESIAN_POINT('Ctrl Pts',(0.00831585952592858,0.0612587666881257,
-0.2608));
#52100=CARTESIAN_POINT('Ctrl Pts',(0.0106237809657182,0.0612936154951835,
-0.2608));
#52101=CARTESIAN_POINT('Ctrl Pts',(0.0129369100215328,0.0612040722239185,
-0.2608));
#52102=CARTESIAN_POINT('Ctrl Pts',(0.0152328715218333,0.0609941762980662,
-0.2608));
#52103=CARTESIAN_POINT('Ctrl Pts',(0.0208062876393118,0.060484656719456,
-0.2608));
#52104=CARTESIAN_POINT('Ctrl Pts',(0.0262953704594572,0.0592700592891648,
-0.2608));
#52105=CARTESIAN_POINT('Ctrl Pts',(0.0315473617407771,0.0573779411784005,
-0.2608));
#52106=CARTESIAN_POINT('Ctrl Pts',(0.0337256011567474,0.0565931938268203,
-0.2608));
#52107=CARTESIAN_POINT('Ctrl Pts',(0.0358639963394174,0.0556903260001544,
-0.2608));
#52108=CARTESIAN_POINT('Ctrl Pts',(0.037936308404479,0.0546778727850125,
-0.2608));
#52109=CARTESIAN_POINT('Ctrl Pts',(0.0396703860429882,0.0538306681047839,
-0.2608));
#52110=CARTESIAN_POINT('Ctrl Pts',(0.0413607927286621,0.0529059149903486,
-0.2608));
#52111=CARTESIAN_POINT('Ctrl Pts',(0.0430016005716766,0.0519049229280611,
-0.2608));
#52112=CARTESIAN_POINT('Ctrl Pts',(0.0469776787705488,0.0494792746517871,
-0.2608));
#52113=CARTESIAN_POINT('Ctrl Pts',(0.0506632023142616,0.0466076377773078,
-0.2608));
#52114=CARTESIAN_POINT('Ctrl Pts',(0.0540354991512064,0.0433644171385233,
-0.2608));
#52115=CARTESIAN_POINT('Ctrl Pts',(0.0556363092948981,0.0418248787325567,
-0.2608));
#52116=CARTESIAN_POINT('Ctrl Pts',(0.0571654283791441,0.0402016121639473,
-0.2608));
#52117=CARTESIAN_POINT('Ctrl Pts',(0.0586117445441614,0.0385124592197734,
-0.2608));
#52118=CARTESIAN_POINT('Ctrl Pts',(0.0616191130766601,0.0350001528971615,
-0.2608));
#52119=CARTESIAN_POINT('Ctrl Pts',(0.0642799176321896,0.03119412357567,
-0.2608));
#52120=CARTESIAN_POINT('Ctrl Pts',(0.0665734050653256,0.0271625612678484,
-0.2608));
#52121=CARTESIAN_POINT('Ctrl Pts',(0.067877037446238,0.0248709964246282,
-0.2608));
#52122=CARTESIAN_POINT('Ctrl Pts',(0.0690618528571677,0.0225062289479046,
-0.2608));
#52123=CARTESIAN_POINT('Ctrl Pts',(0.0701224224214427,0.0200787123815737,
-0.2608));
#52124=CARTESIAN_POINT('Ctrl Pts',(0.0710336990934438,0.0179929093448766,
-0.2608));
#52125=CARTESIAN_POINT('Ctrl Pts',(0.0718509983303909,0.0158652248358311,
-0.2608));
#52126=CARTESIAN_POINT('Ctrl Pts',(0.0725692291932556,0.0137105298517765,
-0.2608));
#52127=CARTESIAN_POINT('Ctrl Pts',(0.0745628323709498,0.00772971366958114,
-0.2608));
#52128=CARTESIAN_POINT('Ctrl Pts',(0.075803672795126,0.00152629816288074,
-0.2608));
#52129=CARTESIAN_POINT('Ctrl Pts',(0.0762256437052851,-0.00475840477433878,
-0.2608));
#52130=CARTESIAN_POINT('Ctrl Pts',(0.0763225129083206,-0.00620114442815519,
-0.2608));
#52131=CARTESIAN_POINT('Ctrl Pts',(0.0763760414501779,-0.00764827653023567,
-0.2608));
#52132=CARTESIAN_POINT('Ctrl Pts',(0.0763850617480247,-0.00909823976109972,
-0.2608));
#52133=CARTESIAN_POINT('Ctrl Pts',(-0.0213170383639359,0.0528823612671139,
-0.2608));
#52134=CARTESIAN_POINT('Ctrl Pts',(-0.0374176429429495,0.0462851352608232,
-0.259090899643908));
#52135=CARTESIAN_POINT('Ctrl Pts',(-0.0541851500158396,0.0276036057596925,
-0.256886440469423));
#52136=CARTESIAN_POINT('Ctrl Pts',(-0.0569449337627208,0.00510999790404281,
-0.254681981294937));
#52137=CARTESIAN_POINT('Ctrl Pts',(-0.0569006472781276,4.53843407899964E-5,
-0.254186622476544));
#52138=CARTESIAN_POINT('Origin',(-8.56069748352724E-18,0.,-0.2608));
#52139=CARTESIAN_POINT('Ctrl Pts',(0.0402078774433248,-0.0657264351496036,
-0.2608));
#52140=CARTESIAN_POINT('Ctrl Pts',(0.03840501184466,-0.0665514984825666,
-0.2608));
#52141=CARTESIAN_POINT('Ctrl Pts',(0.0365711080731641,-0.0673004738245226,
-0.2608));
#52142=CARTESIAN_POINT('Ctrl Pts',(0.0347085406762429,-0.0679692337987251,
-0.2608));
#52143=CARTESIAN_POINT('Ctrl Pts',(0.0307574340573107,-0.0693878895557819,
-0.2608));
#52144=CARTESIAN_POINT('Ctrl Pts',(0.0266771922882156,-0.0704462029385511,
-0.2608));
#52145=CARTESIAN_POINT('Ctrl Pts',(0.0225169930888394,-0.0711480516798359,
-0.2608));
#52146=CARTESIAN_POINT('Ctrl Pts',(0.0198505558885779,-0.0715978944645273,
-0.2608));
#52147=CARTESIAN_POINT('Ctrl Pts',(0.0171522231608511,-0.071900485047978,
-0.2608));
#52148=CARTESIAN_POINT('Ctrl Pts',(0.0144480376767543,-0.0720557703186741,
-0.2608));
#52149=CARTESIAN_POINT('Ctrl Pts',(0.00963208362378582,-0.0723323218840802,
-0.2608));
#52150=CARTESIAN_POINT('Ctrl Pts',(0.00478610537538501,-0.0721447195123662,
-0.2608));
#52151=CARTESIAN_POINT('Ctrl Pts',(-1.05853114393216E-5,-0.0714926725959277,
-0.2608));
#52152=CARTESIAN_POINT('Ctrl Pts',(-0.00238310774834253,-0.0711701594217067,
-0.2608));
#52153=CARTESIAN_POINT('Ctrl Pts',(-0.00473375942598217,-0.0707350657326281,
-0.2608));
#52154=CARTESIAN_POINT('Ctrl Pts',(-0.00705229055096965,-0.0701887458749432,
-0.2608));
#52155=CARTESIAN_POINT('Ctrl Pts',(-0.0125588485324242,-0.0688912252420131,
-0.2608));
#52156=CARTESIAN_POINT('Ctrl Pts',(-0.0178885952542184,-0.0669682018600874,
-0.2608));
#52157=CARTESIAN_POINT('Ctrl Pts',(-0.0228999257528728,-0.0644110854236582,
-0.2608));
#52158=CARTESIAN_POINT('Ctrl Pts',(-0.025169697563011,-0.063252895836241,
-0.2608));
#52159=CARTESIAN_POINT('Ctrl Pts',(-0.0273743491726387,-0.0619629919729461,
-0.2608));
#52160=CARTESIAN_POINT('Ctrl Pts',(-0.0294830145775675,-0.0605508776511837,
-0.2608));
#52161=CARTESIAN_POINT('Ctrl Pts',(-0.0308512530790306,-0.0596346065448305,
-0.2608));
#52162=CARTESIAN_POINT('Ctrl Pts',(-0.0321808825317382,-0.0586660307193501,
-0.2608));
#52163=CARTESIAN_POINT('Ctrl Pts',(-0.0334682470120922,-0.057644991907959,
-0.2608));
#52164=CARTESIAN_POINT('Ctrl Pts',(-0.0359842192458113,-0.0556495156165024,
-0.2608));
#52165=CARTESIAN_POINT('Ctrl Pts',(-0.038339074216195,-0.0534537337051408,
-0.2608));
#52166=CARTESIAN_POINT('Ctrl Pts',(-0.0405192125274857,-0.0510820654044234,
-0.2608));
#52167=CARTESIAN_POINT('Ctrl Pts',(-0.0420374569847095,-0.0494304398019148,
-0.2608));
#52168=CARTESIAN_POINT('Ctrl Pts',(-0.0434720119114289,-0.0476918885002342,
-0.2608));
#52169=CARTESIAN_POINT('Ctrl Pts',(-0.0448131165510465,-0.0458794128670817,
-0.2608));
#52170=CARTESIAN_POINT('Ctrl Pts',(-0.0480480989637234,-0.0415073999581369,
-0.2608));
#52171=CARTESIAN_POINT('Ctrl Pts',(-0.0507184359083405,-0.0367411900030903,
-0.2608));
#52172=CARTESIAN_POINT('Ctrl Pts',(-0.0527554915500067,-0.031704765903902,
-0.2608));
#52173=CARTESIAN_POINT('Ctrl Pts',(-0.053582489134558,-0.0296600939373581,
-0.2608));
#52174=CARTESIAN_POINT('Ctrl Pts',(-0.0543045290184477,-0.027570818899863,
-0.2608));
#52175=CARTESIAN_POINT('Ctrl Pts',(-0.0549145299902943,-0.0254455356779525,
-0.2608));
#52176=CARTESIAN_POINT('Ctrl Pts',(-0.0555211088708353,-0.0233321752456298,
-0.2608));
#52177=CARTESIAN_POINT('Ctrl Pts',(-0.0560143434956106,-0.0211916487578729,
-0.2608));
#52178=CARTESIAN_POINT('Ctrl Pts',(-0.0563884430537062,-0.0190366683982668,
-0.2608));
#52179=CARTESIAN_POINT('Ctrl Pts',(-0.0572390829420659,-0.0141366031272891,
-0.2608));
#52180=CARTESIAN_POINT('Ctrl Pts',(-0.0574789625599653,-0.00915308502654382,
-0.2608));
#52181=CARTESIAN_POINT('Ctrl Pts',(-0.0570218042902053,-0.00419471110367059,
-0.2608));
#52182=CARTESIAN_POINT('Ctrl Pts',(-0.0569755453692129,-0.00369298327171148,
-0.2608));
#52183=CARTESIAN_POINT('Ctrl Pts',(-0.0569221102450288,-0.00319153404867538,
-0.2608));
#52184=CARTESIAN_POINT('Ctrl Pts',(-0.0568613829974075,-0.00269049226390562,
-0.2608));
#52185=CARTESIAN_POINT('Origin',(0.,0.,-0.2608));
#52186=CARTESIAN_POINT('Origin',(0.,0.,-0.348563377523455));
#52187=CARTESIAN_POINT('Ctrl Pts',(-0.0768390318326847,-0.00363576842162216,
-0.272347005383793));
#52188=CARTESIAN_POINT('Ctrl Pts',(-0.0756297895989668,-0.0291921272748137,
-0.270494304666896));
#52189=CARTESIAN_POINT('Ctrl Pts',(-0.0457312801109783,-0.0785610117659347,
-0.266788903233103));
#52190=CARTESIAN_POINT('Ctrl Pts',(0.0413956021036019,-0.0810270855071931,
-0.261230801082413));
#52191=CARTESIAN_POINT('Ctrl Pts',(0.0904399304474149,-0.00914058864406769,
-0.255672698931724));
#52192=CARTESIAN_POINT('Ctrl Pts',(0.0567595801668698,0.0710354832281223,
-0.250114596781034));
#52193=CARTESIAN_POINT('Ctrl Pts',(-0.0289404735607893,0.0862080259423309,
-0.244556494630344));
#52194=CARTESIAN_POINT('Ctrl Pts',(-0.0881160803218006,0.0224199181711109,
-0.238998392479654));
#52195=CARTESIAN_POINT('Ctrl Pts',(-0.0666187715640982,-0.0618859388776004,
-0.233440290328965));
#52196=CARTESIAN_POINT('Ctrl Pts',(0.0158864875285228,-0.0895304755589645,
-0.227882188178275));
#52197=CARTESIAN_POINT('Ctrl Pts',(0.0838413116627435,-0.035190906921961,
-0.222324086027586));
#52198=CARTESIAN_POINT('Ctrl Pts',(0.0750265680498761,0.051370415775385,
-0.216765983876896));
#52199=CARTESIAN_POINT('Ctrl Pts',(-0.00248916725037839,0.0908939972417645,
-0.211207881726206));
#52200=CARTESIAN_POINT('Ctrl Pts',(-0.0777251105279176,0.0471876862083083,
-0.205649779575517));
#52201=CARTESIAN_POINT('Ctrl Pts',(-0.0817903384063056,-0.0397269904622011,
-0.200091677424827));
#52202=CARTESIAN_POINT('Ctrl Pts',(-0.0109620003647857,-0.0902647609758724,
-0.194533575274138));
#52203=CARTESIAN_POINT('Ctrl Pts',(0.0699038979380953,-0.0581492190409055,
-0.188975473123448));
#52204=CARTESIAN_POINT('Ctrl Pts',(0.0867605397727151,0.0272121099867807,
-0.183417370972758));
#52205=CARTESIAN_POINT('Ctrl Pts',(0.0241726471960079,0.0876559919191793,
-0.177859268822068));
#52206=CARTESIAN_POINT('Ctrl Pts',(-0.0605495384751532,0.0678354068241687,
-0.172301166671379));
#52207=CARTESIAN_POINT('Ctrl Pts',(-0.089827992392664,-0.0141004027750951,
-0.166743064520689));
#52208=CARTESIAN_POINT('Ctrl Pts',(-0.0368531383870938,-0.0831248197956735,
-0.16118496237));
#52209=CARTESIAN_POINT('Ctrl Pts',(0.0498672352218698,-0.0760338624070072,
-0.15562686021931));
#52210=CARTESIAN_POINT('Ctrl Pts',(0.0909253969415671,0.000679450155712014,
-0.15006875806862));
#52211=CARTESIAN_POINT('Ctrl Pts',(0.0487253867959945,0.0767706071593588,
-0.144510655917931));
#52212=CARTESIAN_POINT('Ctrl Pts',(-0.0380912730997252,0.0825647887933278,
-0.138952553767241));
#52213=CARTESIAN_POINT('Ctrl Pts',(-0.0900286820059233,0.0127564043178722,
-0.133394451616551));
#52214=CARTESIAN_POINT('Ctrl Pts',(-0.0595290195873821,-0.0687327088728571,
-0.127836349465862));
#52215=CARTESIAN_POINT('Ctrl Pts',(0.0254799164407697,-0.0872849547153862,
-0.122278247315172));
#52216=CARTESIAN_POINT('Ctrl Pts',(0.0871575130564052,-0.0259124931070623,
-0.116720145164483));
#52217=CARTESIAN_POINT('Ctrl Pts',(0.0690270987348237,0.059187406728918,
-0.111162043013793));
#52218=CARTESIAN_POINT('Ctrl Pts',(-0.0123097505872792,0.0900908409118009,
-0.105603940863103));
#52219=CARTESIAN_POINT('Ctrl Pts',(-0.0823748575161993,0.0385002841254505,
-0.100045838712414));
#52220=CARTESIAN_POINT('Ctrl Pts',(-0.0770113205312119,-0.0483440410168286,
-0.0944877365617239));
#52221=CARTESIAN_POINT('Ctrl Pts',(-0.0011303800594704,-0.0909209130646338,
-0.0889296344110343));
#52222=CARTESIAN_POINT('Ctrl Pts',(0.0757855973555288,-0.0502437046352328,
-0.0833715322603447));
#52223=CARTESIAN_POINT('Ctrl Pts',(0.08330659564698,0.0364404122882757,
-0.0778134301096549));
#52224=CARTESIAN_POINT('Ctrl Pts',(0.0145456849523811,0.0897569845586842,
-0.0722553279589654));
#52225=CARTESIAN_POINT('Ctrl Pts',(-0.0675341875961008,0.0608851709532417,
-0.0666972258082757));
#52226=CARTESIAN_POINT('Ctrl Pts',(-0.0877749673282103,-0.0237375187986834,
-0.0611391236575861));
#52227=CARTESIAN_POINT('Ctrl Pts',(-0.0276417441681033,-0.0866247049612507,
-0.0555810215068964));
#52228=CARTESIAN_POINT('Ctrl Pts',(0.0578012067159718,-0.0701910676190134,
-0.0500229193562068));
#52229=CARTESIAN_POINT('Ctrl Pts',(0.0903191709888608,0.0105135099606726,
-0.0444648172055171));
#52230=CARTESIAN_POINT('Ctrl Pts',(0.040129952376398,0.0815936092947214,
-0.0389067150548276));
#52231=CARTESIAN_POINT('Ctrl Pts',(-0.0467974742865224,0.0779557101338933,
-0.0333486129041377));
#52232=CARTESIAN_POINT('Ctrl Pts',(-0.0908884149763414,0.00294461710323904,
-0.0277905107534482));
#52233=CARTESIAN_POINT('Ctrl Pts',(-0.0517269167922935,-0.0747797826777754,
-0.0222324086027586));
#52234=CARTESIAN_POINT('Ctrl Pts',(0.034746178488519,-0.0839978241416842,
-0.0166743064520689));
#52235=CARTESIAN_POINT('Ctrl Pts',(0.0895054655926491,-0.0163632542103587,
-0.0111162043013793));
#52236=CARTESIAN_POINT('Ctrl Pts',(0.0621043605299032,0.0663794467696732,
-0.0055581021506896));
#52237=CARTESIAN_POINT('Ctrl Pts',(0.00622569384473579,0.0808287455412029,
-0.00185270071689654));
#52238=CARTESIAN_POINT('Ctrl Pts',(-0.0186000842079609,0.0746424309120273,
0.));
#52239=CARTESIAN_POINT('Ctrl Pts',(-0.070179815554259,-0.00332067636904975,
-0.268498003589195));
#52240=CARTESIAN_POINT('Ctrl Pts',(-0.0690753716941705,-0.0266622061590246,
-0.266645302872298));
#52241=CARTESIAN_POINT('Ctrl Pts',(-0.0417680015833232,-0.0717525609574906,
-0.262939901438505));
#52242=CARTESIAN_POINT('Ctrl Pts',(0.0378080729428522,-0.0740049136508661,
-0.257381799287816));
#52243=CARTESIAN_POINT('Ctrl Pts',(0.0826019990902562,-0.00834842409902848,
-0.251823697137126));
#52244=CARTESIAN_POINT('Ctrl Pts',(0.0518405395284235,0.0648792285880511,
-0.246265594986436));
#52245=CARTESIAN_POINT('Ctrl Pts',(-0.0264323618883129,0.0787368504733823,
-0.240707492835747));
#52246=CARTESIAN_POINT('Ctrl Pts',(-0.0804795442739791,0.020476907171556,
-0.235149390685057));
#52247=CARTESIAN_POINT('Ctrl Pts',(-0.0608452890322729,-0.0565226249243906,
-0.229591288534368));
#52248=CARTESIAN_POINT('Ctrl Pts',(0.0145096930292469,-0.0817713616550351,
-0.224033186383678));
#52249=CARTESIAN_POINT('Ctrl Pts',(0.0765752463036064,-0.0321411045671164,
-0.218475084232988));
#52250=CARTESIAN_POINT('Ctrl Pts',(0.0685244280390537,0.0469184243746368,
-0.212916982082298));
#52251=CARTESIAN_POINT('Ctrl Pts',(-0.00227344481507348,0.0830167144128823,
-0.207358879931609));
#52252=CARTESIAN_POINT('Ctrl Pts',(-0.0709891026823609,0.0430981889743522,
-0.201800777780919));
#52253=CARTESIAN_POINT('Ctrl Pts',(-0.0747020196190622,-0.0362840706951381,
-0.19624267563023));
#52254=CARTESIAN_POINT('Ctrl Pts',(-0.0100119840835777,-0.0824420105933897,
-0.19068457347954));
#52255=CARTESIAN_POINT('Ctrl Pts',(0.0638457115714528,-0.0531097460441851,
-0.185126471328851));
#52256=CARTESIAN_POINT('Ctrl Pts',(0.0792414809688833,0.0248537860793576,
-0.179568369178161));
#52257=CARTESIAN_POINT('Ctrl Pts',(0.0220777368117798,0.0800593292027518,
-0.174010267027471));
#52258=CARTESIAN_POINT('Ctrl Pts',(-0.0553020429946938,0.0619564852057811,
-0.168452164876781));
#52259=CARTESIAN_POINT('Ctrl Pts',(-0.0820430943410844,-0.0128783984180293,
-0.162894062726092));
#52260=CARTESIAN_POINT('Ctrl Pts',(-0.0336592795733491,-0.0759208488459889,
-0.157335960575402));
#52261=CARTESIAN_POINT('Ctrl Pts',(0.0455455162122831,-0.0694444257343166,
-0.151777858424713));
#52262=CARTESIAN_POINT('Ctrl Pts',(0.0830453928733998,0.00062056594765577,
-0.146219756274023));
#52263=CARTESIAN_POINT('Ctrl Pts',(0.0445026255093734,0.0701173208710384,
-0.140661654123333));
#52264=CARTESIAN_POINT('Ctrl Pts',(-0.0347901119601109,0.0754093526504762,
-0.135103551972643));
#52265=CARTESIAN_POINT('Ctrl Pts',(-0.0822263912893447,0.0116508769151748,
-0.129545449821954));
#52266=CARTESIAN_POINT('Ctrl Pts',(-0.0543699668661269,-0.0627760230210226,
-0.123987347671264));
#52267=CARTESIAN_POINT('Ctrl Pts',(0.0232717122210088,-0.0797204477527267,
-0.118429245520575));
#52268=CARTESIAN_POINT('Ctrl Pts',(0.0796040507614075,-0.0236667998467815,
-0.112871143369885));
#52269=CARTESIAN_POINT('Ctrl Pts',(0.0630448997327806,0.054057959715254,
-0.107313041219195));
#52270=CARTESIAN_POINT('Ctrl Pts',(-0.0112429322068414,0.0822831632247203,
-0.101754939068506));
#52271=CARTESIAN_POINT('Ctrl Pts',(-0.0752358816725248,0.0351636762497748,
-0.0961968369178162));
#52272=CARTESIAN_POINT('Ctrl Pts',(-0.0703371729388632,-0.0441543288715073,
-0.0906387347671264));
#52273=CARTESIAN_POINT('Ctrl Pts',(-0.001032416236745,-0.0830412975894191,
-0.0850806326164368));
#52274=CARTESIAN_POINT('Ctrl Pts',(0.0692176764494058,-0.0458893590921511,
-0.0795225304657471));
#52275=CARTESIAN_POINT('Ctrl Pts',(0.0760868711840199,0.0332823221755449,
-0.0739644283150575));
#52276=CARTESIAN_POINT('Ctrl Pts',(0.0132850904380373,0.0819782403655364,
-0.0684063261643678));
#52277=CARTESIAN_POINT('Ctrl Pts',(-0.0616813709915206,0.0556085880518666,
-0.0628482240136782));
#52278=CARTESIAN_POINT('Ctrl Pts',(-0.0801679936674403,-0.0216803185994695,
-0.0572901218629885));
#52279=CARTESIAN_POINT('Ctrl Pts',(-0.0252461862291492,-0.0791174182134443,
-0.0517320197122989));
#52280=CARTESIAN_POINT('Ctrl Pts',(0.0527918940334048,-0.0641079938355434,
-0.0461739175616093));
#52281=CARTESIAN_POINT('Ctrl Pts',(0.0824917051898045,0.00960236187611665,
-0.0406158154109197));
#52282=CARTESIAN_POINT('Ctrl Pts',(0.0366521101164998,0.0745223399375795,
-0.0350577132602299));
#52283=CARTESIAN_POINT('Ctrl Pts',(-0.0427417945736834,0.0711997174887719,
-0.0294996111095404));
#52284=CARTESIAN_POINT('Ctrl Pts',(-0.0830116159317013,0.00268942333413568,
-0.0239415089588506));
#52285=CARTESIAN_POINT('Ctrl Pts',(-0.0472440294091458,-0.068299030197847,
-0.0183834068081611));
#52286=CARTESIAN_POINT('Ctrl Pts',(0.031734918301019,-0.0767181947068073,
-0.0128253046574713));
#52287=CARTESIAN_POINT('Ctrl Pts',(0.0817485191649469,-0.0149451409649585,
-0.0072672025067818));
#52288=CARTESIAN_POINT('Ctrl Pts',(0.0567221171733953,0.0606267052015075,
-0.00170910035609209));
#52289=CARTESIAN_POINT('Ctrl Pts',(0.00568614720019127,0.0738237627188692,
0.00199630107770095));
#52290=CARTESIAN_POINT('Ctrl Pts',(-0.0169881172091128,0.0681735819542088,
0.0038490017945975));
#52291=CARTESIAN_POINT('Ctrl Pts',(-0.0635205992758333,-0.00300558431647733,
-0.264649001794598));
#52292=CARTESIAN_POINT('Ctrl Pts',(-0.0625209537893743,-0.0241322850432355,
-0.262796301077701));
#52293=CARTESIAN_POINT('Ctrl Pts',(-0.0378047230556681,-0.0649441101490466,
-0.259090899643908));
#52294=CARTESIAN_POINT('Ctrl Pts',(0.0342205437821026,-0.066982741794539,
-0.253532797493218));
#52295=CARTESIAN_POINT('Ctrl Pts',(0.0747640677330976,-0.00755625955398936,
-0.247974695342529));
#52296=CARTESIAN_POINT('Ctrl Pts',(0.0469214988899772,0.05872297394798,
-0.242416593191839));
#52297=CARTESIAN_POINT('Ctrl Pts',(-0.0239242502158365,0.0712656750044335,
-0.23685849104115));
#52298=CARTESIAN_POINT('Ctrl Pts',(-0.0728430082261576,0.0185338961720012,
-0.231300388890459));
#52299=CARTESIAN_POINT('Ctrl Pts',(-0.0550718065004475,-0.051159310971181,
-0.22574228673977));
#52300=CARTESIAN_POINT('Ctrl Pts',(0.013132898529971,-0.0740122477511057,
-0.22018418458908));
#52301=CARTESIAN_POINT('Ctrl Pts',(0.0693091809444694,-0.0290913022122718,
-0.214626082438391));
#52302=CARTESIAN_POINT('Ctrl Pts',(0.0620222880282312,0.0424664329738887,
-0.209067980287701));
#52303=CARTESIAN_POINT('Ctrl Pts',(-0.00205772237976836,0.075139431584,
-0.203509878137012));
#52304=CARTESIAN_POINT('Ctrl Pts',(-0.0642530948368044,0.0390086917403961,
-0.197951775986322));
#52305=CARTESIAN_POINT('Ctrl Pts',(-0.0676137008318185,-0.032841150928075,
-0.192393673835632));
#52306=CARTESIAN_POINT('Ctrl Pts',(-0.00906196780236982,-0.074619260210907,
-0.186835571684942));
#52307=CARTESIAN_POINT('Ctrl Pts',(0.0577875252048107,-0.0480702730474647,
-0.181277469534253));
#52308=CARTESIAN_POINT('Ctrl Pts',(0.0717224221650512,0.0224954621719345,
-0.175719367383563));
#52309=CARTESIAN_POINT('Ctrl Pts',(0.019982826427552,0.0724626664863242,
-0.170161265232874));
#52310=CARTESIAN_POINT('Ctrl Pts',(-0.0500545475142344,0.0560775635873935,
-0.164603163082184));
#52311=CARTESIAN_POINT('Ctrl Pts',(-0.0742581962895047,-0.0116563940609636,
-0.159045060931494));
#52312=CARTESIAN_POINT('Ctrl Pts',(-0.0304654207596044,-0.0687168778963044,
-0.153486958780805));
#52313=CARTESIAN_POINT('Ctrl Pts',(0.0412237972026965,-0.062854989061626,
-0.147928856630115));
#52314=CARTESIAN_POINT('Ctrl Pts',(0.0751653888052323,0.000561681739599467,
-0.142370754479425));
#52315=CARTESIAN_POINT('Ctrl Pts',(0.0402798642227526,0.0634640345827179,
-0.136812652328736));
#52316=CARTESIAN_POINT('Ctrl Pts',(-0.0314889508204967,0.0682539165076246,
-0.131254550178046));
#52317=CARTESIAN_POINT('Ctrl Pts',(-0.074424100572766,0.0105453495124774,
-0.125696448027356));
#52318=CARTESIAN_POINT('Ctrl Pts',(-0.0492109141448716,-0.0568193371691881,
-0.120138345876667));
#52319=CARTESIAN_POINT('Ctrl Pts',(0.0210635080012477,-0.0721559407900673,
-0.114580243725977));
#52320=CARTESIAN_POINT('Ctrl Pts',(0.0720505884664099,-0.0214211065865007,
-0.109022141575287));
#52321=CARTESIAN_POINT('Ctrl Pts',(0.0570627007307374,0.0489285127015899,
-0.103464039424598));
#52322=CARTESIAN_POINT('Ctrl Pts',(-0.0101761138264036,0.0744754855376397,
-0.0979059372739082));
#52323=CARTESIAN_POINT('Ctrl Pts',(-0.0680969058288505,0.0318270683740991,
-0.0923478351232185));
#52324=CARTESIAN_POINT('Ctrl Pts',(-0.0636630253465145,-0.039964616726186,
-0.086789732972529));
#52325=CARTESIAN_POINT('Ctrl Pts',(-0.00093445241401957,-0.0751616821142043,
-0.0812316308218392));
#52326=CARTESIAN_POINT('Ctrl Pts',(0.0626497555432827,-0.0415350135490693,
-0.0756735286711497));
#52327=CARTESIAN_POINT('Ctrl Pts',(0.0688671467210598,0.030124232062814,
-0.0701154265204599));
#52328=CARTESIAN_POINT('Ctrl Pts',(0.0120244959236936,0.0741994961723886,
-0.0645573243697704));
#52329=CARTESIAN_POINT('Ctrl Pts',(-0.0558285543869405,0.0503320051504913,
-0.0589992222190807));
#52330=CARTESIAN_POINT('Ctrl Pts',(-0.0725610200066702,-0.0196231184002554,
-0.0534411200683911));
#52331=CARTESIAN_POINT('Ctrl Pts',(-0.0228506282901951,-0.0716101314656381,
-0.0478830179177014));
#52332=CARTESIAN_POINT('Ctrl Pts',(0.0477825813508377,-0.0580249200520732,
-0.0423249157670118));
#52333=CARTESIAN_POINT('Ctrl Pts',(0.0746642393907483,0.00869121379156067,
-0.0367668136163221));
#52334=CARTESIAN_POINT('Ctrl Pts',(0.0331742678566015,0.0674510705804377,
-0.0312087114656325));
#52335=CARTESIAN_POINT('Ctrl Pts',(-0.0386861148608444,0.0644437248436505,
-0.0256506093149428));
#52336=CARTESIAN_POINT('Ctrl Pts',(-0.0751348168870612,0.00243422956503228,
-0.0200925071642532));
#52337=CARTESIAN_POINT('Ctrl Pts',(-0.0427611420259981,-0.0618182777179186,
-0.0145344050135636));
#52338=CARTESIAN_POINT('Ctrl Pts',(0.0287236581135189,-0.0694385652719304,
-0.00897630286287385));
#52339=CARTESIAN_POINT('Ctrl Pts',(0.0739915727372447,-0.0135270277195584,
-0.00341820071218429));
#52340=CARTESIAN_POINT('Ctrl Pts',(0.0513398738168874,0.0548739636333419,
0.0021399014385054));
#52341=CARTESIAN_POINT('Ctrl Pts',(0.00514660055564675,0.0668187798965355,
0.00584530287229846));
#52342=CARTESIAN_POINT('Ctrl Pts',(-0.0153761502102646,0.0617047329963903,
0.007698003589195));
#52343=CARTESIAN_POINT('Ctrl Pts',(-0.0568613829974075,-0.00269049226390492,
-0.2608));
#52344=CARTESIAN_POINT('Ctrl Pts',(-0.0559665358845781,-0.0216023639274464,
-0.258947299283104));
#52345=CARTESIAN_POINT('Ctrl Pts',(-0.0338414445280129,-0.0581356593406026,
-0.255241897849311));
#52346=CARTESIAN_POINT('Ctrl Pts',(0.030633014621353,-0.0599605699382118,
-0.249683795698621));
#52347=CARTESIAN_POINT('Ctrl Pts',(0.0669261363759389,-0.00676409500895024,
-0.244125693547931));
#52348=CARTESIAN_POINT('Ctrl Pts',(0.0420024582515309,0.0525667193079089,
-0.238567591397241));
#52349=CARTESIAN_POINT('Ctrl Pts',(-0.0214161385433601,0.0637944995354849,
-0.233009489246552));
#52350=CARTESIAN_POINT('Ctrl Pts',(-0.0652064721783362,0.0165908851724463,
-0.227451387095862));
#52351=CARTESIAN_POINT('Ctrl Pts',(-0.0492983239686221,-0.0457959970179712,
-0.221893284945172));
#52352=CARTESIAN_POINT('Ctrl Pts',(0.011756104030695,-0.0662531338471764,
-0.216335182794483));
#52353=CARTESIAN_POINT('Ctrl Pts',(0.0620431155853323,-0.0260414998574271,
-0.210777080643793));
#52354=CARTESIAN_POINT('Ctrl Pts',(0.0555201480174088,0.0380144415731405,
-0.205218978493103));
#52355=CARTESIAN_POINT('Ctrl Pts',(-0.00184199994446337,0.0672621487551179,
-0.199660876342414));
#52356=CARTESIAN_POINT('Ctrl Pts',(-0.0575170869912477,0.0349191945064401,
-0.194102774191724));
#52357=CARTESIAN_POINT('Ctrl Pts',(-0.060525382044575,-0.029398231161012,
-0.188544672041035));
#52358=CARTESIAN_POINT('Ctrl Pts',(-0.00811195152116181,-0.0667965098284243,
-0.182986569890345));
#52359=CARTESIAN_POINT('Ctrl Pts',(0.0517293388381684,-0.0430308000507443,
-0.177428467739655));
#52360=CARTESIAN_POINT('Ctrl Pts',(0.0642033633612193,0.0201371382645114,
-0.171870365588966));
#52361=CARTESIAN_POINT('Ctrl Pts',(0.0178879160433239,0.0648660037698966,
-0.166312263438276));
#52362=CARTESIAN_POINT('Ctrl Pts',(-0.0448070520337749,0.0501986419690058,
-0.160754161287587));
#52363=CARTESIAN_POINT('Ctrl Pts',(-0.0664732982379252,-0.0104343897038979,
-0.155196059136897));
#52364=CARTESIAN_POINT('Ctrl Pts',(-0.0272715619458597,-0.0615129069466198,
-0.149637956986207));
#52365=CARTESIAN_POINT('Ctrl Pts',(0.0369020781931099,-0.0562655523889355,
-0.144079854835517));
#52366=CARTESIAN_POINT('Ctrl Pts',(0.0672853847370649,0.000502797531543261,
-0.138521752684828));
#52367=CARTESIAN_POINT('Ctrl Pts',(0.0360571029361317,0.0568107482943974,
-0.132963650534138));
#52368=CARTESIAN_POINT('Ctrl Pts',(-0.0281877896808826,0.0610984803647731,
-0.127405548383449));
#52369=CARTESIAN_POINT('Ctrl Pts',(-0.0666218098561871,0.00943982210977994,
-0.121847446232759));
#52370=CARTESIAN_POINT('Ctrl Pts',(-0.0440518614236164,-0.0508626513173536,
-0.116289344082069));
#52371=CARTESIAN_POINT('Ctrl Pts',(0.0188553037814868,-0.0645914338274078,
-0.110731241931379));
#52372=CARTESIAN_POINT('Ctrl Pts',(0.0644971261714122,-0.0191754133262199,
-0.10517313978069));
#52373=CARTESIAN_POINT('Ctrl Pts',(0.0510805017286943,0.0437990656879258,
-0.0996150376300002));
#52374=CARTESIAN_POINT('Ctrl Pts',(-0.00910929544596579,0.0666678078505591,
-0.0940569354793109));
#52375=CARTESIAN_POINT('Ctrl Pts',(-0.060957929985176,0.0284904604984234,
-0.0884988333286209));
#52376=CARTESIAN_POINT('Ctrl Pts',(-0.0569888777541658,-0.0357749045808647,
-0.0829407311779316));
#52377=CARTESIAN_POINT('Ctrl Pts',(-0.000836488591294147,-0.0672820666389896,
-0.0773826290272417));
#52378=CARTESIAN_POINT('Ctrl Pts',(0.0560818346371597,-0.0371806680059875,
-0.0718245268765522));
#52379=CARTESIAN_POINT('Ctrl Pts',(0.0616474222580996,0.0269661419500831,
-0.0662664247258625));
#52380=CARTESIAN_POINT('Ctrl Pts',(0.0107639014093499,0.0664207519792408,
-0.0607083225751728));
#52381=CARTESIAN_POINT('Ctrl Pts',(-0.0499757377823604,0.045055422249116,
-0.0551502204244832));
#52382=CARTESIAN_POINT('Ctrl Pts',(-0.0649540463459001,-0.0175659182010413,
-0.0495921182737936));
#52383=CARTESIAN_POINT('Ctrl Pts',(-0.0204550703512412,-0.0641028447178318,
-0.0440340161231039));
#52384=CARTESIAN_POINT('Ctrl Pts',(0.0427732686682708,-0.0519418462686033,
-0.0384759139724143));
#52385=CARTESIAN_POINT('Ctrl Pts',(0.0668367735916919,0.00778006570700472,
-0.0329178118217246));
#52386=CARTESIAN_POINT('Ctrl Pts',(0.0296964255967034,0.0603798012232959,
-0.027359709671035));
#52387=CARTESIAN_POINT('Ctrl Pts',(-0.0346304351480055,0.0576877321985291,
-0.0218016075203453));
#52388=CARTESIAN_POINT('Ctrl Pts',(-0.067258017842421,0.00217903579592891,
-0.0162435053696557));
#52389=CARTESIAN_POINT('Ctrl Pts',(-0.0382782546428504,-0.0553375252379902,
-0.0106854032189661));
#52390=CARTESIAN_POINT('Ctrl Pts',(0.0257123979260188,-0.0621589358370536,
-0.00512730106827636));
#52391=CARTESIAN_POINT('Ctrl Pts',(0.0662346263095425,-0.0121089144741581,
0.000430801082413216));
#52392=CARTESIAN_POINT('Ctrl Pts',(0.0459576304603796,0.0491212220651762,
0.00598890323310289));
#52393=CARTESIAN_POINT('Ctrl Pts',(0.00460705391110222,0.0598137970742019,
0.00969430466689595));
#52394=CARTESIAN_POINT('Ctrl Pts',(-0.0137641832114165,0.0552358840385719,
0.0115470053837925));
#52395=CARTESIAN_POINT('',(-0.0186000842079609,0.0746424309120273,0.));
#52396=CARTESIAN_POINT('Ctrl Pts',(0.0551371004056304,-0.0145210214852671,
-1.38777878078145E-17));
#52397=CARTESIAN_POINT('Ctrl Pts',(0.0557629658139121,-0.0131629595984533,
-1.70794074384518E-17));
#52398=CARTESIAN_POINT('Ctrl Pts',(0.0563303031086066,-0.0117815320725005,
-9.07936409284168E-17));
#52399=CARTESIAN_POINT('Ctrl Pts',(0.0568367962277587,-0.0103798601340677,
-8.84708972748172E-17));
#52400=CARTESIAN_POINT('Ctrl Pts',(0.0579324744939598,-0.00734767386892008,
-8.52714485894961E-17));
#52401=CARTESIAN_POINT('Ctrl Pts',(0.0587439674756155,-0.00422113471852991,
-5.91471153565421E-17));
#52402=CARTESIAN_POINT('Ctrl Pts',(0.0592872651796402,-0.00103525413784158,
-5.72458747072346E-17));
#52403=CARTESIAN_POINT('Ctrl Pts',(0.0596976535666042,0.00137125040448081,
-5.58097429556742E-17));
#52404=CARTESIAN_POINT('Ctrl Pts',(0.0599540529871003,0.00381003129288719,
1.13065255910782E-17));
#52405=CARTESIAN_POINT('Ctrl Pts',(0.0600621304227767,0.00625467285507289,
8.67361737988404E-18));
#52406=CARTESIAN_POINT('Ctrl Pts',(0.0602044555315557,0.00947397459077743,
5.20639089344986E-18));
#52407=CARTESIAN_POINT('Ctrl Pts',(0.0600908652691288,0.0127087915017173,
-8.32645063813673E-17));
#52408=CARTESIAN_POINT('Ctrl Pts',(0.0597334763142803,0.0159280092132275,
-7.97972798949331E-17));
#52409=CARTESIAN_POINT('Ctrl Pts',(0.0594787929043323,0.0182220961820871,
-7.73264562932321E-17));
#52410=CARTESIAN_POINT('Ctrl Pts',(0.0591000457868719,0.0205057594111829,
-8.69735018148149E-17));
#52411=CARTESIAN_POINT('Ctrl Pts',(0.058604046859906,0.022757306393025,
-6.93889390390723E-17));
#52412=CARTESIAN_POINT('Ctrl Pts',(0.0574000150098037,0.0282229115198812,
-2.67026094906683E-17));
#52413=CARTESIAN_POINT('Ctrl Pts',(0.0555070346110573,0.0335164792257551,
6.58435981494048E-17));
#52414=CARTESIAN_POINT('Ctrl Pts',(0.0529715910690817,0.0384899104332707,
7.89299181569447E-17));
#52415=CARTESIAN_POINT('Ctrl Pts',(0.0519200213889706,0.0405526301812588,
8.43574408433455E-17));
#52416=CARTESIAN_POINT('Ctrl Pts',(0.0507562550697398,0.0425610151284201,
-1.69820238630303E-17));
#52417=CARTESIAN_POINT('Ctrl Pts',(0.0494920486484344,0.0444901026849085,
-1.90819582357449E-17));
#52418=CARTESIAN_POINT('Ctrl Pts',(0.0484341874343681,0.0461043223804862,
-2.08391389362553E-17));
#52419=CARTESIAN_POINT('Ctrl Pts',(0.0473048627097976,0.0476654962951114,
-6.98109579163092E-18));
#52420=CARTESIAN_POINT('Ctrl Pts',(0.0461061165839465,0.0491679074422925,
7.80625564189563E-18));
#52421=CARTESIAN_POINT('Ctrl Pts',(0.0432012619200474,0.0528086166248848,
4.35741111720786E-17));
#52422=CARTESIAN_POINT('Ctrl Pts',(0.0398903515469501,0.0561051665186203,
5.00499939764873E-17));
#52423=CARTESIAN_POINT('Ctrl Pts',(0.0362500452078145,0.0590443888276636,
4.33680868994202E-17));
#52424=CARTESIAN_POINT('Ctrl Pts',(0.0345220116191685,0.0604396216463748,
4.01962220095754E-17));
#52425=CARTESIAN_POINT('Ctrl Pts',(0.0327198952772362,0.0617532349568333,
5.64086294081436E-17));
#52426=CARTESIAN_POINT('Ctrl Pts',(0.0308627900046538,0.0629764406192712,
4.85722573273506E-17));
#52427=CARTESIAN_POINT('Ctrl Pts',(0.0270012557184676,0.0655198885725436,
3.22778555419218E-17));
#52428=CARTESIAN_POINT('Ctrl Pts',(0.0228917503466347,0.0676826925597205,
-5.93019284099973E-17));
#52429=CARTESIAN_POINT('Ctrl Pts',(0.0186045273957792,0.0694528091662133,
-6.93889390390723E-17));
#52430=CARTESIAN_POINT('Ctrl Pts',(0.0161676416790297,0.070458955085096,
-7.51224622097737E-17));
#52431=CARTESIAN_POINT('Ctrl Pts',(0.0136730221737058,0.0713380460700889,
1.16527597969391E-16));
#52432=CARTESIAN_POINT('Ctrl Pts',(0.0111317204605169,0.0720860061518305,
1.28803218091278E-16));
#52433=CARTESIAN_POINT('Ctrl Pts',(0.00894815151273096,0.0727286777402524,
1.39350829488168E-16));
#52434=CARTESIAN_POINT('Ctrl Pts',(0.00673480985803829,0.0732728638103404,
3.27324123811703E-17));
#52435=CARTESIAN_POINT('Ctrl Pts',(0.00450708731124494,0.0737153773487098,
3.16587034365767E-17));
#52436=CARTESIAN_POINT('Ctrl Pts',(-0.00167643327094307,0.0749436683566466,
2.8678394525249E-17));
#52437=CARTESIAN_POINT('Ctrl Pts',(-0.00798645148332497,0.0753972328474082,
-6.20569042812721E-17));
#52438=CARTESIAN_POINT('Ctrl Pts',(-0.0142744840883698,0.0750281955405284,
-6.74915852372227E-17));
#52439=CARTESIAN_POINT('Ctrl Pts',(-0.0157179901554196,0.0749434778514024,
-6.87391924659289E-17));
#52440=CARTESIAN_POINT('Ctrl Pts',(-0.0171604219804116,0.0748152105438323,
-2.91779109939374E-18));
#52441=CARTESIAN_POINT('Ctrl Pts',(-0.0186000842079609,0.0746424309120273,
0.));
#52442=CARTESIAN_POINT('Ctrl Pts',(-0.0186000842079609,0.0746424309120273,
0.));
#52443=CARTESIAN_POINT('Ctrl Pts',(0.00622569384473562,0.0808287455412029,
-0.00185270071689653));
#52444=CARTESIAN_POINT('Ctrl Pts',(0.0341650271873191,0.0736040961554381,
-0.00370540143379305));
#52445=CARTESIAN_POINT('Ctrl Pts',(0.0527015447024019,0.0562013212992173,
-0.00555810215068958));
#52446=CARTESIAN_POINT('Ctrl Pts',(0.071238062217485,0.0387985464429963,
-0.00741080286758614));
#52447=CARTESIAN_POINT('Ctrl Pts',(0.0803717639050671,0.0112176461163188,
-0.00926350358448272));
#52448=CARTESIAN_POINT('Ctrl Pts',(0.0758120668981698,-0.0138452323689076,
-0.0111162043013793));
#52449=CARTESIAN_POINT('Ctrl Pts',(0.0712523698912725,-0.0389081108541336,
-0.0129689050182758));
#52450=CARTESIAN_POINT('Ctrl Pts',(0.0529992741898961,-0.0614529674979086,
-0.0148216057351723));
#52451=CARTESIAN_POINT('Ctrl Pts',(0.0294605437924059,-0.0711890555758115,
-0.0166743064520688));
#52452=CARTESIAN_POINT('Ctrl Pts',(0.00592181339491531,-0.0809251436537147,
-0.0185270071689654));
#52453=CARTESIAN_POINT('Ctrl Pts',(-0.0229025516986893,-0.0778524631657451,
-0.020379707885862));
#52454=CARTESIAN_POINT('Ctrl Pts',(-0.0438416506094996,-0.063362056291591,
-0.0222324086027586));
#52455=CARTESIAN_POINT('Ctrl Pts',(-0.0641021519188406,-0.0493412567960065,
-0.0240250667042551));
#52456=CARTESIAN_POINT('Ctrl Pts',(-0.0769801991262393,-0.0246307939408685,
-0.0258177248057515));
#52457=CARTESIAN_POINT('Ctrl Pts',(-0.0770493699172285,1.64405594954022E-5,
-0.027610382907248));
#52458=CARTESIAN_POINT('Origin',(-0.0288,-0.1152,0.0585));
#52459=CARTESIAN_POINT('',(0.0288,-0.1152,0.13));
#52460=CARTESIAN_POINT('',(-0.0288,-0.1152,0.13));
#52461=CARTESIAN_POINT('',(-0.0144,-0.1152,0.13));
#52462=CARTESIAN_POINT('',(0.0288,-0.1152,0.0585));
#52463=CARTESIAN_POINT('',(0.0288,-0.1152,0.0585));
#52464=CARTESIAN_POINT('',(-0.0288,-0.1152,0.0585));
#52465=CARTESIAN_POINT('',(-0.0288,-0.1152,0.0585));
#52466=CARTESIAN_POINT('',(-0.0288,-0.1152,0.0585));
#52467=CARTESIAN_POINT('Origin',(0.0288,-0.1152,0.0585));
#52468=CARTESIAN_POINT('',(0.0288,0.1152,0.13));
#52469=CARTESIAN_POINT('',(0.0288,0.0288,0.13));
#52470=CARTESIAN_POINT('',(0.0288,-0.0576,0.13));
#52471=CARTESIAN_POINT('',(0.0288,0.1152,0.0585));
#52472=CARTESIAN_POINT('',(0.0288,0.1152,0.0585));
#52473=CARTESIAN_POINT('',(0.0288,0.0288,0.0585));
#52474=CARTESIAN_POINT('',(0.0288,-0.1152,0.0585));
#52475=CARTESIAN_POINT('',(0.0288,0.0288,0.0585));
#52476=CARTESIAN_POINT('Origin',(-0.0288,0.1152,0.0585));
#52477=CARTESIAN_POINT('',(-0.0288,0.0288,0.13));
#52478=CARTESIAN_POINT('',(-0.0288,0.1152,0.13));
#52479=CARTESIAN_POINT('',(-0.0288,0.0576,0.13));
#52480=CARTESIAN_POINT('',(-0.0288,0.0288,0.0585));
#52481=CARTESIAN_POINT('',(-0.0288,0.0288,0.0585));
#52482=CARTESIAN_POINT('',(-0.0288,0.1152,0.0585));
#52483=CARTESIAN_POINT('',(-0.0288,0.1152,0.0585));
#52484=CARTESIAN_POINT('',(-0.0288,0.1152,0.0585));
#52485=CARTESIAN_POINT('Origin',(-0.0288,0.1152,0.0585));
#52486=CARTESIAN_POINT('',(-0.0288,-0.0288,0.13));
#52487=CARTESIAN_POINT('',(-0.0288,0.0576,0.13));
#52488=CARTESIAN_POINT('',(-0.0288,-0.0288,0.0585));
#52489=CARTESIAN_POINT('',(-0.0288,0.1152,0.0585));
#52490=CARTESIAN_POINT('',(-0.0288,-0.0288,0.0585));
#52491=CARTESIAN_POINT('Origin',(0.0288,0.1152,0.0585));
#52492=CARTESIAN_POINT('',(0.0144,0.1152,0.13));
#52493=CARTESIAN_POINT('',(0.0288,0.1152,0.0585));
#52494=CARTESIAN_POINT('Origin',(0.0288,-0.1152,0.0585));
#52495=CARTESIAN_POINT('',(0.0288,-0.0288,0.13));
#52496=CARTESIAN_POINT('',(0.0288,-0.0576,0.13));
#52497=CARTESIAN_POINT('',(0.0288,-0.0288,0.0585));
#52498=CARTESIAN_POINT('',(0.0288,-0.0288,0.0585));
#52499=CARTESIAN_POINT('',(0.0288,-0.1152,0.0585));
#52500=CARTESIAN_POINT('Origin',(0.,0.,0.13));
#52501=CARTESIAN_POINT('',(-0.1275,-1.56142466891288E-17,0.13));
#52502=CARTESIAN_POINT('Origin',(0.,0.,0.13));
#52503=CARTESIAN_POINT('',(-0.1152,-0.0288,0.13));
#52504=CARTESIAN_POINT('',(-0.0576,-0.0288,0.13));
#52505=CARTESIAN_POINT('',(-0.1152,0.0288,0.13));
#52506=CARTESIAN_POINT('',(-0.1152,0.0144,0.13));
#52507=CARTESIAN_POINT('',(0.0576,0.0288,0.13));
#52508=CARTESIAN_POINT('',(0.1152,0.0288,0.13));
#52509=CARTESIAN_POINT('',(0.0576,0.0288,0.13));
#52510=CARTESIAN_POINT('',(0.1152,-0.0288,0.13));
#52511=CARTESIAN_POINT('',(0.1152,-0.0144,0.13));
#52512=CARTESIAN_POINT('',(-0.0576,-0.0288,0.13));
#52513=CARTESIAN_POINT('Origin',(-0.1152,-0.0288,0.0585));
#52514=CARTESIAN_POINT('',(-0.1152,-0.0288,0.0585));
#52515=CARTESIAN_POINT('',(-0.1152,-0.0288,0.0585));
#52516=CARTESIAN_POINT('',(-0.1152,-0.0288,0.0585));
#52517=CARTESIAN_POINT('Origin',(0.1152,0.0288,0.0585));
#52518=CARTESIAN_POINT('',(-0.1152,0.0288,0.0585));
#52519=CARTESIAN_POINT('',(-0.1152,0.0288,0.0585));
#52520=CARTESIAN_POINT('',(0.1152,0.0288,0.0585));
#52521=CARTESIAN_POINT('Origin',(0.1152,0.0288,0.0585));
#52522=CARTESIAN_POINT('',(0.1152,0.0288,0.0585));
#52523=CARTESIAN_POINT('',(0.1152,0.0288,0.0585));
#52524=CARTESIAN_POINT('',(0.1152,0.0288,0.0585));
#52525=CARTESIAN_POINT('Origin',(-0.1152,-0.0288,0.0585));
#52526=CARTESIAN_POINT('',(0.1152,-0.0288,0.0585));
#52527=CARTESIAN_POINT('',(0.1152,-0.0288,0.0585));
#52528=CARTESIAN_POINT('',(-0.1152,-0.0288,0.0585));
#52529=CARTESIAN_POINT('Origin',(-0.1152,0.0288,0.0585));
#52530=CARTESIAN_POINT('',(-0.1152,0.0288,0.0585));
#52531=CARTESIAN_POINT('Origin',(0.1152,-0.0288,0.0585));
#52532=CARTESIAN_POINT('',(0.1152,-0.0288,0.0585));
#52533=CARTESIAN_POINT('Origin',(0.,0.,0.0585));
#52534=CARTESIAN_POINT('Origin',(0.0608,0.,-0.3));
#52535=CARTESIAN_POINT('',(-0.0608,-7.44585253881591E-18,-0.3));
#52536=CARTESIAN_POINT('Origin',(0.,0.,-0.3));
#52537=CARTESIAN_POINT('Origin',(0.,0.,-0.2904));
#52538=CARTESIAN_POINT('',(-0.0704,-8.62151346599737E-18,-0.2904));
#52539=CARTESIAN_POINT('Origin',(0.,0.,-0.1404));
#52540=CARTESIAN_POINT('Origin',(0.,0.,0.));
#52541=CARTESIAN_POINT('Origin',(0.16,0.,0.));
#52542=CARTESIAN_POINT('',(-0.16,-1.95943487863577E-17,0.));
#52543=CARTESIAN_POINT('Origin',(0.,0.,0.));
#52544=CARTESIAN_POINT('Origin',(0.,0.,0.039));
#52545=CARTESIAN_POINT('',(-0.16,-1.95943487863577E-17,0.078));
#52546=CARTESIAN_POINT('Origin',(0.,0.,0.078));
#52547=CARTESIAN_POINT('',(-0.16,-1.95943487863577E-17,0.039));
#52548=CARTESIAN_POINT('Origin',(0.,0.,0.104));
#52549=CARTESIAN_POINT('',(-0.14375,-1.76042977377432E-17,0.104));
#54978=UNCERTAINTY_MEASURE_WITH_UNIT(LENGTH_MEASURE(0.001),#55003,
'DISTANCE_ACCURACY_VALUE',
'Maximum model space distance between geometric entities at asserted c
onnectivities');
#54980=UNCERTAINTY_MEASURE_WITH_UNIT(LENGTH_MEASURE(0.001),#55003,
'DISTANCE_ACCURACY_VALUE',
'Maximum model space distance between geometric entities at asserted c
onnectivities');
#55000=(
GEOMETRIC_REPRESENTATION_CONTEXT(3)
GLOBAL_UNCERTAINTY_ASSIGNED_CONTEXT((#54978))
GLOBAL_UNIT_ASSIGNED_CONTEXT((#55003,#55005,#55006))
REPRESENTATION_CONTEXT('','3D')
);
#55002=(
GEOMETRIC_REPRESENTATION_CONTEXT(3)
GLOBAL_UNCERTAINTY_ASSIGNED_CONTEXT((#54980))
GLOBAL_UNIT_ASSIGNED_CONTEXT((#55003,#55005,#55006))
REPRESENTATION_CONTEXT('','3D')
);
#55003=(
LENGTH_UNIT()
NAMED_UNIT(*)
SI_UNIT(.CENTI.,.METRE.)
);
#55005=(
NAMED_UNIT(*)
PLANE_ANGLE_UNIT()
SI_UNIT($,.RADIAN.)
);
#55006=(
NAMED_UNIT(*)
SI_UNIT($,.STERADIAN.)
SOLID_ANGLE_UNIT()
);
#55026=SHAPE_DEFINITION_REPRESENTATION(#55047,#55122);
#55047=PRODUCT_DEFINITION_SHAPE('',$,#55144);
#55122=SHAPE_REPRESENTATION('',(#27025),#55000);
#55124=PRODUCT_DEFINITION_CONTEXT('part definition',#55189,'design');
#55144=PRODUCT_DEFINITION('2026-10-18-23-37-02-926',
'18_ISO_7045_M1.6x3_A2',#55165,#55124);
#55165=PRODUCT_DEFINITION_FORMATION('',$,#55210);
#55189=APPLICATION_CONTEXT(
'Core Data for Automotive Mechanical Design Process');
#55190=PRODUCT_CONTEXT('part definition',#55189,'mechanical');
#55210=PRODUCT('2026-10-18-23-37-02-926','18_ISO_7045_M1.6x3_A2',$,(#55190));
#55394=COLOUR_RGB('Off White',0.89,0.88,0.83);
#55395=FILL_AREA_STYLE_COLOUR('',#55394);
#55396=FILL_AREA_STYLE('',(#55395));
#55397=SURFACE_STYLE_FILL_AREA(#55396);
#55398=SURFACE_SIDE_STYLE('',(#55397));
#55399=SURFACE_STYLE_USAGE(.BOTH.,#55398);
#55400=PRESENTATION_STYLE_ASSIGNMENT((#55399));
ENDSEC;
END-ISO-10303-21;
